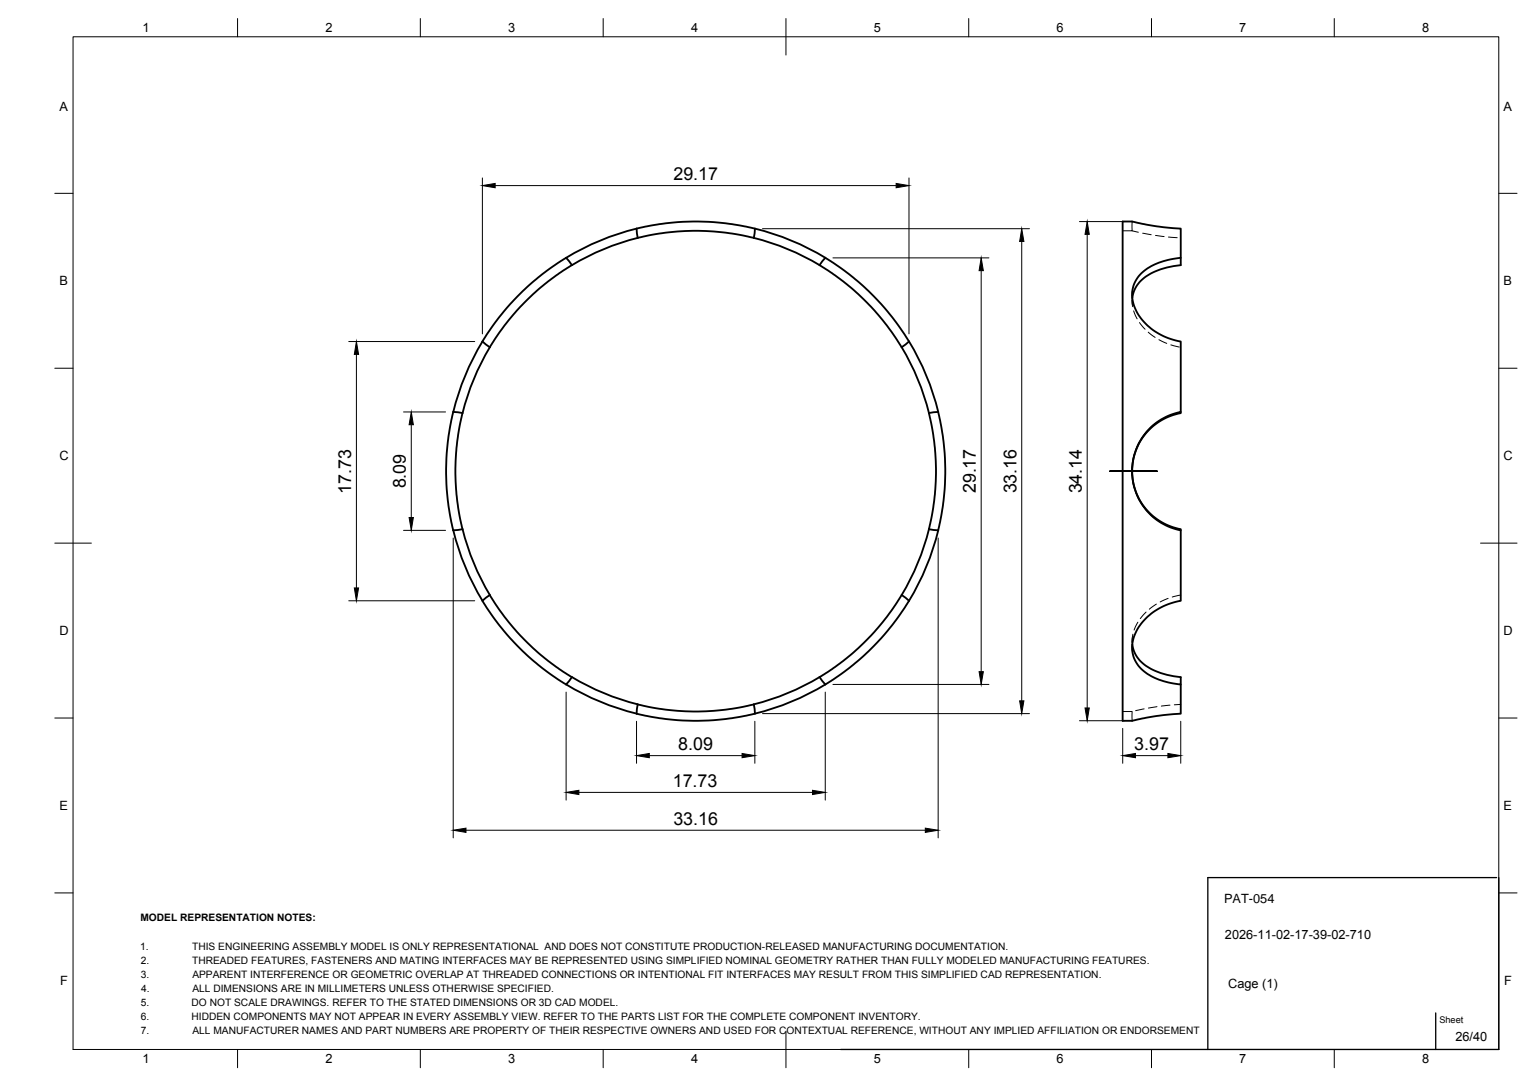
ISO-10303-21;
HEADER;
/* Generated by software containing ST-Developer
 * from STEP Tools, Inc. (www.steptools.com) 
 */

FILE_DESCRIPTION(
/* description */ ('PAT-054'),
/* implementation_level */ '2;1');

FILE_NAME(
/* name */ 'Cage (1).step',
/* time_stamp */ '2026-10-29T16:38:13-07:00',
/* author */ (''),
/* organization */ (''),
/* preprocessor_version */ 'ST-DEVELOPER v20.2',
/* originating_system */ 'Autodesk Translation Framework v15.17.0.0',
/* authorisation */ '');

FILE_SCHEMA (('AUTOMOTIVE_DESIGN { 1 0 10303 214 3 1 1 }'));
ENDSEC;

DATA;
#10=MECHANICAL_DESIGN_GEOMETRIC_PRESENTATION_REPRESENTATION('',(#930),#33981);
#417=B_SPLINE_CURVE_WITH_KNOTS('',3,(#19899,#19900,#19901,#19902,#19903,
#19904,#19905,#19906,#19907,#19908,#19909,#19910,#19911,#19912,#19913,#19914,
#19915,#19916,#19917,#19918,#19919,#19920),.UNSPECIFIED.,.F.,.F.,(4,2,2,
2,2,2,2,2,2,2,4),(0.0789094028588958,0.210573405340968,0.315860108011452,
0.421146810681936,0.522142632548711,0.623138454415485,0.72413427628226,
0.825130098149035,0.930416800819519,1.03570350349,1.16736750597208),
 .UNSPECIFIED.);
#418=B_SPLINE_CURVE_WITH_KNOTS('',3,(#19924,#19925,#19926,#19927,#19928,
#19929,#19930,#19931,#19932,#19933,#19934,#19935,#19936,#19937,#19938,#19939,
#19940,#19941,#19942,#19943,#19944,#19945),.UNSPECIFIED.,.F.,.F.,(4,2,2,
2,2,2,2,2,2,2,4),(0.0774793363974613,0.142088896491891,0.284177792983782,
0.411119756996526,0.514392970548519,0.617666184100513,0.720939397652506,
0.8242126112045,0.951154575217244,1.09324347170913,1.15785303180356),
 .UNSPECIFIED.);
#419=B_SPLINE_CURVE_WITH_KNOTS('',3,(#19951,#19952,#19953,#19954,#19955,
#19956,#19957,#19958,#19959,#19960,#19961,#19962,#19963,#19964,#19965,#19966,
#19967,#19968,#19969,#19970,#19971,#19972),.UNSPECIFIED.,.F.,.F.,(4,2,2,
2,2,2,2,2,2,2,4),(0.0774793363974613,0.142088896491891,0.284177792983782,
0.411119756996525,0.514392970548519,0.617666184100513,0.720939397652506,
0.8242126112045,0.951154575217243,1.09324347170913,1.15785303180356),
 .UNSPECIFIED.);
#420=B_SPLINE_CURVE_WITH_KNOTS('',3,(#19976,#19977,#19978,#19979,#19980,
#19981,#19982,#19983,#19984,#19985,#19986,#19987,#19988,#19989,#19990,#19991,
#19992,#19993,#19994,#19995,#19996,#19997),.UNSPECIFIED.,.F.,.F.,(4,2,2,
2,2,2,2,2,2,2,4),(0.0774793363974614,0.142088896491891,0.284177792983781,
0.411119756996525,0.514392970548519,0.617666184100512,0.720939397652506,
0.824212611204499,0.951154575217243,1.09324347170913,1.15785303180356),
 .UNSPECIFIED.);
#421=B_SPLINE_CURVE_WITH_KNOTS('',3,(#20001,#20002,#20003,#20004,#20005,
#20006,#20007,#20008,#20009,#20010,#20011,#20012),.UNSPECIFIED.,.F.,.F.,
(4,2,2,2,2,4),(0.0774793363974613,0.142088896491891,0.284177792983781,0.411119756996525,
0.514392970548519,0.617666184100512),.UNSPECIFIED.);
#422=B_SPLINE_CURVE_WITH_KNOTS('',3,(#20017,#20018,#20019,#20020,#20021,
#20022,#20023,#20024,#20025,#20026,#20027,#20028),.UNSPECIFIED.,.F.,.F.,
(4,2,2,2,2,4),(0.617666184100512,0.720939397652506,0.824212611204499,0.951154575217243,
1.09324347170913,1.15785303180356),.UNSPECIFIED.);
#423=B_SPLINE_CURVE_WITH_KNOTS('',3,(#20032,#20033,#20034,#20035,#20036,
#20037,#20038,#20039,#20040,#20041,#20042,#20043,#20044,#20045,#20046,#20047,
#20048,#20049,#20050,#20051,#20052,#20053),.UNSPECIFIED.,.F.,.F.,(4,2,2,
2,2,2,2,2,2,2,4),(0.0774793363974613,0.142088896491891,0.284177792983782,
0.411119756996526,0.514392970548519,0.617666184100513,0.720939397652507,
0.8242126112045,0.951154575217245,1.09324347170914,1.15785303180356),
 .UNSPECIFIED.);
#424=B_SPLINE_CURVE_WITH_KNOTS('',3,(#20057,#20058,#20059,#20060,#20061,
#20062,#20063,#20064,#20065,#20066,#20067,#20068,#20069,#20070,#20071,#20072,
#20073,#20074,#20075,#20076,#20077,#20078),.UNSPECIFIED.,.F.,.F.,(4,2,2,
2,2,2,2,2,2,2,4),(0.0774793363974613,0.142088896491891,0.284177792983782,
0.411119756996526,0.514392970548519,0.617666184100513,0.720939397652506,
0.824212611204499,0.951154575217243,1.09324347170913,1.15785303180356),
 .UNSPECIFIED.);
#425=B_SPLINE_CURVE_WITH_KNOTS('',3,(#20082,#20083,#20084,#20085,#20086,
#20087,#20088,#20089,#20090,#20091,#20092,#20093,#20094,#20095,#20096,#20097,
#20098,#20099,#20100,#20101,#20102,#20103),.UNSPECIFIED.,.F.,.F.,(4,2,2,
2,2,2,2,2,2,2,4),(0.0774793363974613,0.142088896491891,0.284177792983782,
0.411119756996526,0.514392970548519,0.617666184100513,0.720939397652506,
0.8242126112045,0.951154575217244,1.09324347170913,1.15785303180356),
 .UNSPECIFIED.);
#426=B_SPLINE_CURVE_WITH_KNOTS('',3,(#20107,#20108,#20109,#20110,#20111,
#20112,#20113,#20114,#20115,#20116,#20117,#20118,#20119,#20120,#20121,#20122,
#20123,#20124,#20125,#20126,#20127,#20128),.UNSPECIFIED.,.F.,.F.,(4,2,2,
2,2,2,2,2,2,2,4),(0.0774793363974613,0.142088896491891,0.284177792983782,
0.411119756996526,0.514392970548519,0.617666184100513,0.720939397652506,
0.8242126112045,0.951154575217243,1.09324347170913,1.15785303180356),
 .UNSPECIFIED.);
#427=B_SPLINE_CURVE_WITH_KNOTS('',3,(#20136,#20137,#20138,#20139,#20140,
#20141,#20142,#20143,#20144,#20145,#20146,#20147,#20148,#20149,#20150,#20151,
#20152,#20153,#20154,#20155,#20156,#20157),.UNSPECIFIED.,.F.,.F.,(4,2,2,
2,2,2,2,2,2,2,4),(0.0789094028588958,0.210573405340968,0.315860108011452,
0.421146810681936,0.522142632548711,0.623138454415485,0.72413427628226,
0.825130098149035,0.930416800819519,1.03570350349,1.16736750597208),
 .UNSPECIFIED.);
#428=B_SPLINE_CURVE_WITH_KNOTS('',3,(#20165,#20166,#20167,#20168,#20169,
#20170,#20171,#20172,#20173,#20174,#20175,#20176,#20177,#20178,#20179,#20180,
#20181,#20182,#20183,#20184,#20185,#20186),.UNSPECIFIED.,.F.,.F.,(4,2,2,
2,2,2,2,2,2,2,4),(0.0789094028588958,0.210573405340969,0.315860108011453,
0.421146810681937,0.522142632548712,0.623138454415486,0.724134276282261,
0.825130098149035,0.930416800819519,1.03570350349,1.16736750597208),
 .UNSPECIFIED.);
#429=B_SPLINE_CURVE_WITH_KNOTS('',3,(#20195,#20196,#20197,#20198,#20199,
#20200,#20201,#20202,#20203,#20204,#20205,#20206),.UNSPECIFIED.,.F.,.F.,
(4,2,2,2,2,4),(0.0789094028588958,0.210573405340968,0.315860108011452,0.421146810681937,
0.522142632548711,0.623138454415486),.UNSPECIFIED.);
#430=B_SPLINE_CURVE_WITH_KNOTS('',3,(#20208,#20209,#20210,#20211,#20212,
#20213,#20214,#20215,#20216,#20217,#20218,#20219),.UNSPECIFIED.,.F.,.F.,
(4,2,2,2,2,4),(0.623138454415486,0.72413427628226,0.825130098149035,0.930416800819519,
1.03570350349,1.16736750597208),.UNSPECIFIED.);
#431=B_SPLINE_CURVE_WITH_KNOTS('',3,(#20226,#20227,#20228,#20229,#20230,
#20231,#20232,#20233,#20234,#20235,#20236,#20237,#20238,#20239,#20240,#20241,
#20242,#20243,#20244,#20245,#20246,#20247),.UNSPECIFIED.,.F.,.F.,(4,2,2,
2,2,2,2,2,2,2,4),(0.0789094028588958,0.210573405340968,0.315860108011452,
0.421146810681936,0.522142632548711,0.623138454415486,0.72413427628226,
0.825130098149035,0.930416800819519,1.03570350349,1.16736750597208),
 .UNSPECIFIED.);
#432=B_SPLINE_CURVE_WITH_KNOTS('',3,(#20255,#20256,#20257,#20258,#20259,
#20260,#20261,#20262,#20263,#20264,#20265,#20266,#20267,#20268,#20269,#20270,
#20271,#20272,#20273,#20274,#20275,#20276),.UNSPECIFIED.,.F.,.F.,(4,2,2,
2,2,2,2,2,2,2,4),(0.0789094028588957,0.210573405340968,0.315860108011452,
0.421146810681936,0.522142632548711,0.623138454415485,0.72413427628226,
0.825130098149035,0.930416800819519,1.03570350349,1.16736750597207),
 .UNSPECIFIED.);
#433=B_SPLINE_CURVE_WITH_KNOTS('',3,(#20284,#20285,#20286,#20287,#20288,
#20289,#20290,#20291,#20292,#20293,#20294,#20295,#20296,#20297,#20298,#20299,
#20300,#20301,#20302,#20303,#20304,#20305),.UNSPECIFIED.,.F.,.F.,(4,2,2,
2,2,2,2,2,2,2,4),(0.0789094028588958,0.210573405340968,0.315860108011452,
0.421146810681936,0.522142632548711,0.623138454415486,0.72413427628226,
0.825130098149035,0.930416800819519,1.03570350349,1.16736750597208),
 .UNSPECIFIED.);
#434=B_SPLINE_CURVE_WITH_KNOTS('',3,(#20314,#20315,#20316,#20317,#20318,
#20319,#20320,#20321,#20322,#20323,#20324,#20325,#20326,#20327,#20328,#20329,
#20330,#20331,#20332,#20333,#20334,#20335),.UNSPECIFIED.,.F.,.F.,(4,2,2,
2,2,2,2,2,2,2,4),(0.0789094028588958,0.210573405340968,0.315860108011452,
0.421146810681936,0.522142632548711,0.623138454415485,0.72413427628226,
0.825130098149035,0.930416800819519,1.03570350349,1.16736750597208),
 .UNSPECIFIED.);
#769=SPHERICAL_SURFACE('',#14058,0.412776);
#770=SPHERICAL_SURFACE('',#14074,0.412776);
#771=SPHERICAL_SURFACE('',#14079,0.412776);
#772=SPHERICAL_SURFACE('',#14084,0.412776);
#773=SPHERICAL_SURFACE('',#14089,0.412776);
#774=SPHERICAL_SURFACE('',#14094,0.412776);
#775=SPHERICAL_SURFACE('',#14099,0.412776);
#776=SPHERICAL_SURFACE('',#14107,0.412776);
#828=SHAPE_REPRESENTATION_RELATIONSHIP('SRR','None',#34203,#872);
#872=ADVANCED_BREP_SHAPE_REPRESENTATION('',(#989),#33951);
#930=STYLED_ITEM('',(#34517),#989);
#989=MANIFOLD_SOLID_BREP('Continuous crown cage',#13041);
#1141=FACE_BOUND('',#2670,.T.);
#1331=PLANE('',#14071);
#1332=PLANE('',#14076);
#1333=PLANE('',#14081);
#1334=PLANE('',#14086);
#1335=PLANE('',#14091);
#1336=PLANE('',#14096);
#1337=PLANE('',#14105);
#1338=PLANE('',#14109);
#1339=PLANE('',#14110);
#1800=FACE_OUTER_BOUND('',#2652,.T.);
#1801=FACE_OUTER_BOUND('',#2653,.T.);
#1802=FACE_OUTER_BOUND('',#2654,.T.);
#1803=FACE_OUTER_BOUND('',#2655,.T.);
#1804=FACE_OUTER_BOUND('',#2656,.T.);
#1805=FACE_OUTER_BOUND('',#2657,.T.);
#1806=FACE_OUTER_BOUND('',#2658,.T.);
#1807=FACE_OUTER_BOUND('',#2659,.T.);
#1808=FACE_OUTER_BOUND('',#2660,.T.);
#1809=FACE_OUTER_BOUND('',#2661,.T.);
#1810=FACE_OUTER_BOUND('',#2662,.T.);
#1811=FACE_OUTER_BOUND('',#2663,.T.);
#1812=FACE_OUTER_BOUND('',#2664,.T.);
#1813=FACE_OUTER_BOUND('',#2665,.T.);
#1814=FACE_OUTER_BOUND('',#2666,.T.);
#1815=FACE_OUTER_BOUND('',#2667,.T.);
#1816=FACE_OUTER_BOUND('',#2668,.T.);
#1817=FACE_OUTER_BOUND('',#2669,.T.);
#1818=FACE_OUTER_BOUND('',#2671,.T.);
#2652=EDGE_LOOP('',(#9505,#9506,#9507,#9508));
#2653=EDGE_LOOP('',(#9509,#9510,#9511,#9512,#9513,#9514,#9515,#9516,#9517,
#9518,#9519,#9520,#9521,#9522,#9523,#9524,#9525,#9526,#9527,#9528));
#2654=EDGE_LOOP('',(#9529,#9530,#9531,#9532));
#2655=EDGE_LOOP('',(#9533,#9534,#9535,#9536));
#2656=EDGE_LOOP('',(#9537,#9538,#9539,#9540));
#2657=EDGE_LOOP('',(#9541,#9542,#9543,#9544));
#2658=EDGE_LOOP('',(#9545,#9546,#9547,#9548));
#2659=EDGE_LOOP('',(#9549,#9550,#9551,#9552,#9553,#9554));
#2660=EDGE_LOOP('',(#9555,#9556,#9557,#9558));
#2661=EDGE_LOOP('',(#9559,#9560,#9561,#9562));
#2662=EDGE_LOOP('',(#9563,#9564,#9565,#9566));
#2663=EDGE_LOOP('',(#9567,#9568,#9569,#9570));
#2664=EDGE_LOOP('',(#9571,#9572,#9573,#9574));
#2665=EDGE_LOOP('',(#9575,#9576,#9577,#9578));
#2666=EDGE_LOOP('',(#9579,#9580,#9581,#9582,#9583,#9584,#9585,#9586,#9587,
#9588,#9589,#9590,#9591,#9592,#9593,#9594,#9595,#9596,#9597,#9598));
#2667=EDGE_LOOP('',(#9599,#9600,#9601,#9602));
#2668=EDGE_LOOP('',(#9603,#9604,#9605,#9606));
#2669=EDGE_LOOP('',(#9607));
#2670=EDGE_LOOP('',(#9608));
#2671=EDGE_LOOP('',(#9609,#9610,#9611,#9612));
#3484=LINE('',#20014,#4418);
#3485=LINE('',#20310,#4419);
#4418=VECTOR('',#16149,1.706752);
#4419=VECTOR('',#16226,1.643248);
#5352=CIRCLE('',#14059,0.405071403305639);
#5353=CIRCLE('',#14060,0.405071403305639);
#5354=CIRCLE('',#14062,1.706752);
#5355=CIRCLE('',#14063,1.706752);
#5356=CIRCLE('',#14064,1.706752);
#5357=CIRCLE('',#14065,1.706752);
#5358=CIRCLE('',#14066,1.706752);
#5359=CIRCLE('',#14067,1.706752);
#5360=CIRCLE('',#14068,1.706752);
#5361=CIRCLE('',#14069,1.706752);
#5362=CIRCLE('',#14070,1.706752);
#5363=CIRCLE('',#14072,1.643248);
#5364=CIRCLE('',#14073,0.405071403305639);
#5365=CIRCLE('',#14075,0.405071403305639);
#5366=CIRCLE('',#14077,1.643248);
#5367=CIRCLE('',#14078,0.405071403305639);
#5368=CIRCLE('',#14080,0.405071403305639);
#5369=CIRCLE('',#14082,1.643248);
#5370=CIRCLE('',#14083,0.405071403305639);
#5371=CIRCLE('',#14085,0.405071403305639);
#5372=CIRCLE('',#14087,1.643248);
#5373=CIRCLE('',#14088,0.405071403305639);
#5374=CIRCLE('',#14090,0.405071403305639);
#5375=CIRCLE('',#14092,1.643248);
#5376=CIRCLE('',#14093,0.405071403305639);
#5377=CIRCLE('',#14095,0.405071403305639);
#5378=CIRCLE('',#14097,1.643248);
#5379=CIRCLE('',#14098,0.405071403305639);
#5380=CIRCLE('',#14100,0.405071403305639);
#5381=CIRCLE('',#14102,1.643248);
#5382=CIRCLE('',#14103,1.643248);
#5383=CIRCLE('',#14104,1.643248);
#5384=CIRCLE('',#14106,0.405071403305639);
#5385=CIRCLE('',#14108,0.405071403305639);
#5926=VERTEX_POINT('',#19897);
#5927=VERTEX_POINT('',#19898);
#5928=VERTEX_POINT('',#19921);
#5929=VERTEX_POINT('',#19923);
#5930=VERTEX_POINT('',#19948);
#5931=VERTEX_POINT('',#19950);
#5932=VERTEX_POINT('',#19973);
#5933=VERTEX_POINT('',#19975);
#5934=VERTEX_POINT('',#19998);
#5935=VERTEX_POINT('',#20000);
#5936=VERTEX_POINT('',#20013);
#5937=VERTEX_POINT('',#20016);
#5938=VERTEX_POINT('',#20029);
#5939=VERTEX_POINT('',#20031);
#5940=VERTEX_POINT('',#20054);
#5941=VERTEX_POINT('',#20056);
#5942=VERTEX_POINT('',#20079);
#5943=VERTEX_POINT('',#20081);
#5944=VERTEX_POINT('',#20104);
#5945=VERTEX_POINT('',#20106);
#5946=VERTEX_POINT('',#20131);
#5947=VERTEX_POINT('',#20135);
#5948=VERTEX_POINT('',#20160);
#5949=VERTEX_POINT('',#20164);
#5950=VERTEX_POINT('',#20189);
#5951=VERTEX_POINT('',#20193);
#5952=VERTEX_POINT('',#20194);
#5953=VERTEX_POINT('',#20221);
#5954=VERTEX_POINT('',#20225);
#5955=VERTEX_POINT('',#20250);
#5956=VERTEX_POINT('',#20254);
#5957=VERTEX_POINT('',#20279);
#5958=VERTEX_POINT('',#20283);
#5959=VERTEX_POINT('',#20308);
#5960=VERTEX_POINT('',#20311);
#5961=VERTEX_POINT('',#20313);
#7252=EDGE_CURVE('',#5926,#5927,#417,.T.);
#7253=EDGE_CURVE('',#5928,#5926,#5352,.T.);
#7254=EDGE_CURVE('',#5929,#5928,#418,.T.);
#7255=EDGE_CURVE('',#5927,#5929,#5353,.T.);
#7256=EDGE_CURVE('',#5930,#5928,#5354,.T.);
#7257=EDGE_CURVE('',#5930,#5931,#419,.T.);
#7258=EDGE_CURVE('',#5932,#5931,#5355,.T.);
#7259=EDGE_CURVE('',#5932,#5933,#420,.T.);
#7260=EDGE_CURVE('',#5934,#5933,#5356,.T.);
#7261=EDGE_CURVE('',#5934,#5935,#421,.T.);
#7262=EDGE_CURVE('',#5935,#5936,#3484,.T.);
#7263=EDGE_CURVE('',#5936,#5936,#5357,.T.);
#7264=EDGE_CURVE('',#5935,#5937,#422,.T.);
#7265=EDGE_CURVE('',#5938,#5937,#5358,.T.);
#7266=EDGE_CURVE('',#5938,#5939,#423,.T.);
#7267=EDGE_CURVE('',#5940,#5939,#5359,.T.);
#7268=EDGE_CURVE('',#5940,#5941,#424,.T.);
#7269=EDGE_CURVE('',#5942,#5941,#5360,.T.);
#7270=EDGE_CURVE('',#5942,#5943,#425,.T.);
#7271=EDGE_CURVE('',#5944,#5943,#5361,.T.);
#7272=EDGE_CURVE('',#5944,#5945,#426,.T.);
#7273=EDGE_CURVE('',#5929,#5945,#5362,.T.);
#7274=EDGE_CURVE('',#5926,#5946,#5363,.T.);
#7275=EDGE_CURVE('',#5946,#5930,#5364,.T.);
#7276=EDGE_CURVE('',#5947,#5946,#427,.T.);
#7277=EDGE_CURVE('',#5931,#5947,#5365,.T.);
#7278=EDGE_CURVE('',#5947,#5948,#5366,.T.);
#7279=EDGE_CURVE('',#5948,#5932,#5367,.T.);
#7280=EDGE_CURVE('',#5949,#5948,#428,.T.);
#7281=EDGE_CURVE('',#5933,#5949,#5368,.T.);
#7282=EDGE_CURVE('',#5949,#5950,#5369,.T.);
#7283=EDGE_CURVE('',#5950,#5934,#5370,.T.);
#7284=EDGE_CURVE('',#5951,#5952,#429,.T.);
#7285=EDGE_CURVE('',#5937,#5951,#5371,.T.);
#7286=EDGE_CURVE('',#5952,#5950,#430,.T.);
#7287=EDGE_CURVE('',#5951,#5953,#5372,.T.);
#7288=EDGE_CURVE('',#5953,#5938,#5373,.T.);
#7289=EDGE_CURVE('',#5954,#5953,#431,.T.);
#7290=EDGE_CURVE('',#5939,#5954,#5374,.T.);
#7291=EDGE_CURVE('',#5954,#5955,#5375,.T.);
#7292=EDGE_CURVE('',#5955,#5940,#5376,.T.);
#7293=EDGE_CURVE('',#5956,#5955,#432,.T.);
#7294=EDGE_CURVE('',#5941,#5956,#5377,.T.);
#7295=EDGE_CURVE('',#5956,#5957,#5378,.T.);
#7296=EDGE_CURVE('',#5957,#5942,#5379,.T.);
#7297=EDGE_CURVE('',#5958,#5957,#433,.T.);
#7298=EDGE_CURVE('',#5943,#5958,#5380,.T.);
#7299=EDGE_CURVE('',#5959,#5959,#5381,.T.);
#7300=EDGE_CURVE('',#5959,#5952,#3485,.T.);
#7301=EDGE_CURVE('',#5960,#5927,#5382,.T.);
#7302=EDGE_CURVE('',#5960,#5961,#434,.T.);
#7303=EDGE_CURVE('',#5958,#5961,#5383,.T.);
#7304=EDGE_CURVE('',#5945,#5960,#5384,.T.);
#7305=EDGE_CURVE('',#5961,#5944,#5385,.T.);
#9505=ORIENTED_EDGE('',*,*,#7252,.F.);
#9506=ORIENTED_EDGE('',*,*,#7253,.F.);
#9507=ORIENTED_EDGE('',*,*,#7254,.F.);
#9508=ORIENTED_EDGE('',*,*,#7255,.F.);
#9509=ORIENTED_EDGE('',*,*,#7254,.T.);
#9510=ORIENTED_EDGE('',*,*,#7256,.F.);
#9511=ORIENTED_EDGE('',*,*,#7257,.T.);
#9512=ORIENTED_EDGE('',*,*,#7258,.F.);
#9513=ORIENTED_EDGE('',*,*,#7259,.T.);
#9514=ORIENTED_EDGE('',*,*,#7260,.F.);
#9515=ORIENTED_EDGE('',*,*,#7261,.T.);
#9516=ORIENTED_EDGE('',*,*,#7262,.T.);
#9517=ORIENTED_EDGE('',*,*,#7263,.F.);
#9518=ORIENTED_EDGE('',*,*,#7262,.F.);
#9519=ORIENTED_EDGE('',*,*,#7264,.T.);
#9520=ORIENTED_EDGE('',*,*,#7265,.F.);
#9521=ORIENTED_EDGE('',*,*,#7266,.T.);
#9522=ORIENTED_EDGE('',*,*,#7267,.F.);
#9523=ORIENTED_EDGE('',*,*,#7268,.T.);
#9524=ORIENTED_EDGE('',*,*,#7269,.F.);
#9525=ORIENTED_EDGE('',*,*,#7270,.T.);
#9526=ORIENTED_EDGE('',*,*,#7271,.F.);
#9527=ORIENTED_EDGE('',*,*,#7272,.T.);
#9528=ORIENTED_EDGE('',*,*,#7273,.F.);
#9529=ORIENTED_EDGE('',*,*,#7253,.T.);
#9530=ORIENTED_EDGE('',*,*,#7274,.T.);
#9531=ORIENTED_EDGE('',*,*,#7275,.T.);
#9532=ORIENTED_EDGE('',*,*,#7256,.T.);
#9533=ORIENTED_EDGE('',*,*,#7276,.F.);
#9534=ORIENTED_EDGE('',*,*,#7277,.F.);
#9535=ORIENTED_EDGE('',*,*,#7257,.F.);
#9536=ORIENTED_EDGE('',*,*,#7275,.F.);
#9537=ORIENTED_EDGE('',*,*,#7277,.T.);
#9538=ORIENTED_EDGE('',*,*,#7278,.T.);
#9539=ORIENTED_EDGE('',*,*,#7279,.T.);
#9540=ORIENTED_EDGE('',*,*,#7258,.T.);
#9541=ORIENTED_EDGE('',*,*,#7280,.F.);
#9542=ORIENTED_EDGE('',*,*,#7281,.F.);
#9543=ORIENTED_EDGE('',*,*,#7259,.F.);
#9544=ORIENTED_EDGE('',*,*,#7279,.F.);
#9545=ORIENTED_EDGE('',*,*,#7281,.T.);
#9546=ORIENTED_EDGE('',*,*,#7282,.T.);
#9547=ORIENTED_EDGE('',*,*,#7283,.T.);
#9548=ORIENTED_EDGE('',*,*,#7260,.T.);
#9549=ORIENTED_EDGE('',*,*,#7284,.F.);
#9550=ORIENTED_EDGE('',*,*,#7285,.F.);
#9551=ORIENTED_EDGE('',*,*,#7264,.F.);
#9552=ORIENTED_EDGE('',*,*,#7261,.F.);
#9553=ORIENTED_EDGE('',*,*,#7283,.F.);
#9554=ORIENTED_EDGE('',*,*,#7286,.F.);
#9555=ORIENTED_EDGE('',*,*,#7285,.T.);
#9556=ORIENTED_EDGE('',*,*,#7287,.T.);
#9557=ORIENTED_EDGE('',*,*,#7288,.T.);
#9558=ORIENTED_EDGE('',*,*,#7265,.T.);
#9559=ORIENTED_EDGE('',*,*,#7289,.F.);
#9560=ORIENTED_EDGE('',*,*,#7290,.F.);
#9561=ORIENTED_EDGE('',*,*,#7266,.F.);
#9562=ORIENTED_EDGE('',*,*,#7288,.F.);
#9563=ORIENTED_EDGE('',*,*,#7290,.T.);
#9564=ORIENTED_EDGE('',*,*,#7291,.T.);
#9565=ORIENTED_EDGE('',*,*,#7292,.T.);
#9566=ORIENTED_EDGE('',*,*,#7267,.T.);
#9567=ORIENTED_EDGE('',*,*,#7293,.F.);
#9568=ORIENTED_EDGE('',*,*,#7294,.F.);
#9569=ORIENTED_EDGE('',*,*,#7268,.F.);
#9570=ORIENTED_EDGE('',*,*,#7292,.F.);
#9571=ORIENTED_EDGE('',*,*,#7294,.T.);
#9572=ORIENTED_EDGE('',*,*,#7295,.T.);
#9573=ORIENTED_EDGE('',*,*,#7296,.T.);
#9574=ORIENTED_EDGE('',*,*,#7269,.T.);
#9575=ORIENTED_EDGE('',*,*,#7270,.F.);
#9576=ORIENTED_EDGE('',*,*,#7296,.F.);
#9577=ORIENTED_EDGE('',*,*,#7297,.F.);
#9578=ORIENTED_EDGE('',*,*,#7298,.F.);
#9579=ORIENTED_EDGE('',*,*,#7299,.F.);
#9580=ORIENTED_EDGE('',*,*,#7300,.T.);
#9581=ORIENTED_EDGE('',*,*,#7286,.T.);
#9582=ORIENTED_EDGE('',*,*,#7282,.F.);
#9583=ORIENTED_EDGE('',*,*,#7280,.T.);
#9584=ORIENTED_EDGE('',*,*,#7278,.F.);
#9585=ORIENTED_EDGE('',*,*,#7276,.T.);
#9586=ORIENTED_EDGE('',*,*,#7274,.F.);
#9587=ORIENTED_EDGE('',*,*,#7252,.T.);
#9588=ORIENTED_EDGE('',*,*,#7301,.F.);
#9589=ORIENTED_EDGE('',*,*,#7302,.T.);
#9590=ORIENTED_EDGE('',*,*,#7303,.F.);
#9591=ORIENTED_EDGE('',*,*,#7297,.T.);
#9592=ORIENTED_EDGE('',*,*,#7295,.F.);
#9593=ORIENTED_EDGE('',*,*,#7293,.T.);
#9594=ORIENTED_EDGE('',*,*,#7291,.F.);
#9595=ORIENTED_EDGE('',*,*,#7289,.T.);
#9596=ORIENTED_EDGE('',*,*,#7287,.F.);
#9597=ORIENTED_EDGE('',*,*,#7284,.T.);
#9598=ORIENTED_EDGE('',*,*,#7300,.F.);
#9599=ORIENTED_EDGE('',*,*,#7255,.T.);
#9600=ORIENTED_EDGE('',*,*,#7273,.T.);
#9601=ORIENTED_EDGE('',*,*,#7304,.T.);
#9602=ORIENTED_EDGE('',*,*,#7301,.T.);
#9603=ORIENTED_EDGE('',*,*,#7272,.F.);
#9604=ORIENTED_EDGE('',*,*,#7305,.F.);
#9605=ORIENTED_EDGE('',*,*,#7302,.F.);
#9606=ORIENTED_EDGE('',*,*,#7304,.F.);
#9607=ORIENTED_EDGE('',*,*,#7263,.T.);
#9608=ORIENTED_EDGE('',*,*,#7299,.T.);
#9609=ORIENTED_EDGE('',*,*,#7298,.T.);
#9610=ORIENTED_EDGE('',*,*,#7303,.T.);
#9611=ORIENTED_EDGE('',*,*,#7305,.T.);
#9612=ORIENTED_EDGE('',*,*,#7271,.T.);
#12067=CYLINDRICAL_SURFACE('',#14061,1.706752);
#12068=CYLINDRICAL_SURFACE('',#14101,1.643248);
#12512=ADVANCED_FACE('',(#1800),#769,.F.);
#12513=ADVANCED_FACE('',(#1801),#12067,.T.);
#12514=ADVANCED_FACE('',(#1802),#1331,.T.);
#12515=ADVANCED_FACE('',(#1803),#770,.F.);
#12516=ADVANCED_FACE('',(#1804),#1332,.T.);
#12517=ADVANCED_FACE('',(#1805),#771,.F.);
#12518=ADVANCED_FACE('',(#1806),#1333,.T.);
#12519=ADVANCED_FACE('',(#1807),#772,.F.);
#12520=ADVANCED_FACE('',(#1808),#1334,.T.);
#12521=ADVANCED_FACE('',(#1809),#773,.F.);
#12522=ADVANCED_FACE('',(#1810),#1335,.T.);
#12523=ADVANCED_FACE('',(#1811),#774,.F.);
#12524=ADVANCED_FACE('',(#1812),#1336,.T.);
#12525=ADVANCED_FACE('',(#1813),#775,.F.);
#12526=ADVANCED_FACE('',(#1814),#12068,.F.);
#12527=ADVANCED_FACE('',(#1815),#1337,.T.);
#12528=ADVANCED_FACE('',(#1816),#776,.F.);
#12529=ADVANCED_FACE('',(#1817,#1141),#1338,.T.);
#12530=ADVANCED_FACE('',(#1818),#1339,.T.);
#13041=CLOSED_SHELL('',(#12512,#12513,#12514,#12515,#12516,#12517,#12518,
#12519,#12520,#12521,#12522,#12523,#12524,#12525,#12526,#12527,#12528,#12529,
#12530));
#14057=AXIS2_PLACEMENT_3D('',#19895,#16133,#16134);
#14058=AXIS2_PLACEMENT_3D('',#19896,#16135,#16136);
#14059=AXIS2_PLACEMENT_3D('',#19922,#16137,#16138);
#14060=AXIS2_PLACEMENT_3D('',#19946,#16139,#16140);
#14061=AXIS2_PLACEMENT_3D('',#19947,#16141,#16142);
#14062=AXIS2_PLACEMENT_3D('',#19949,#16143,#16144);
#14063=AXIS2_PLACEMENT_3D('',#19974,#16145,#16146);
#14064=AXIS2_PLACEMENT_3D('',#19999,#16147,#16148);
#14065=AXIS2_PLACEMENT_3D('',#20015,#16150,#16151);
#14066=AXIS2_PLACEMENT_3D('',#20030,#16152,#16153);
#14067=AXIS2_PLACEMENT_3D('',#20055,#16154,#16155);
#14068=AXIS2_PLACEMENT_3D('',#20080,#16156,#16157);
#14069=AXIS2_PLACEMENT_3D('',#20105,#16158,#16159);
#14070=AXIS2_PLACEMENT_3D('',#20129,#16160,#16161);
#14071=AXIS2_PLACEMENT_3D('',#20130,#16162,#16163);
#14072=AXIS2_PLACEMENT_3D('',#20132,#16164,#16165);
#14073=AXIS2_PLACEMENT_3D('',#20133,#16166,#16167);
#14074=AXIS2_PLACEMENT_3D('',#20134,#16168,#16169);
#14075=AXIS2_PLACEMENT_3D('',#20158,#16170,#16171);
#14076=AXIS2_PLACEMENT_3D('',#20159,#16172,#16173);
#14077=AXIS2_PLACEMENT_3D('',#20161,#16174,#16175);
#14078=AXIS2_PLACEMENT_3D('',#20162,#16176,#16177);
#14079=AXIS2_PLACEMENT_3D('',#20163,#16178,#16179);
#14080=AXIS2_PLACEMENT_3D('',#20187,#16180,#16181);
#14081=AXIS2_PLACEMENT_3D('',#20188,#16182,#16183);
#14082=AXIS2_PLACEMENT_3D('',#20190,#16184,#16185);
#14083=AXIS2_PLACEMENT_3D('',#20191,#16186,#16187);
#14084=AXIS2_PLACEMENT_3D('',#20192,#16188,#16189);
#14085=AXIS2_PLACEMENT_3D('',#20207,#16190,#16191);
#14086=AXIS2_PLACEMENT_3D('',#20220,#16192,#16193);
#14087=AXIS2_PLACEMENT_3D('',#20222,#16194,#16195);
#14088=AXIS2_PLACEMENT_3D('',#20223,#16196,#16197);
#14089=AXIS2_PLACEMENT_3D('',#20224,#16198,#16199);
#14090=AXIS2_PLACEMENT_3D('',#20248,#16200,#16201);
#14091=AXIS2_PLACEMENT_3D('',#20249,#16202,#16203);
#14092=AXIS2_PLACEMENT_3D('',#20251,#16204,#16205);
#14093=AXIS2_PLACEMENT_3D('',#20252,#16206,#16207);
#14094=AXIS2_PLACEMENT_3D('',#20253,#16208,#16209);
#14095=AXIS2_PLACEMENT_3D('',#20277,#16210,#16211);
#14096=AXIS2_PLACEMENT_3D('',#20278,#16212,#16213);
#14097=AXIS2_PLACEMENT_3D('',#20280,#16214,#16215);
#14098=AXIS2_PLACEMENT_3D('',#20281,#16216,#16217);
#14099=AXIS2_PLACEMENT_3D('',#20282,#16218,#16219);
#14100=AXIS2_PLACEMENT_3D('',#20306,#16220,#16221);
#14101=AXIS2_PLACEMENT_3D('',#20307,#16222,#16223);
#14102=AXIS2_PLACEMENT_3D('',#20309,#16224,#16225);
#14103=AXIS2_PLACEMENT_3D('',#20312,#16227,#16228);
#14104=AXIS2_PLACEMENT_3D('',#20336,#16229,#16230);
#14105=AXIS2_PLACEMENT_3D('',#20337,#16231,#16232);
#14106=AXIS2_PLACEMENT_3D('',#20338,#16233,#16234);
#14107=AXIS2_PLACEMENT_3D('',#20339,#16235,#16236);
#14108=AXIS2_PLACEMENT_3D('',#20340,#16237,#16238);
#14109=AXIS2_PLACEMENT_3D('',#20341,#16239,#16240);
#14110=AXIS2_PLACEMENT_3D('',#20342,#16241,#16242);
#16133=DIRECTION('axis',(0.,0.,1.));
#16134=DIRECTION('refdir',(1.,0.,0.));
#16135=DIRECTION('center_axis',(0.,0.,1.));
#16136=DIRECTION('ref_axis',(1.,0.,0.));
#16137=DIRECTION('center_axis',(0.,-1.,0.));
#16138=DIRECTION('ref_axis',(0.,0.,-1.));
#16139=DIRECTION('center_axis',(0.,-1.,0.));
#16140=DIRECTION('ref_axis',(0.,0.,-1.));
#16141=DIRECTION('center_axis',(0.,1.,0.));
#16142=DIRECTION('ref_axis',(1.,0.,0.));
#16143=DIRECTION('center_axis',(0.,1.,0.));
#16144=DIRECTION('ref_axis',(1.,0.,0.));
#16145=DIRECTION('center_axis',(0.,1.,0.));
#16146=DIRECTION('ref_axis',(1.,0.,0.));
#16147=DIRECTION('center_axis',(0.,1.,0.));
#16148=DIRECTION('ref_axis',(1.,0.,0.));
#16149=DIRECTION('',(0.,-1.,0.));
#16150=DIRECTION('center_axis',(0.,-1.,0.));
#16151=DIRECTION('ref_axis',(1.,0.,0.));
#16152=DIRECTION('center_axis',(0.,1.,0.));
#16153=DIRECTION('ref_axis',(1.,0.,0.));
#16154=DIRECTION('center_axis',(0.,1.,0.));
#16155=DIRECTION('ref_axis',(1.,0.,0.));
#16156=DIRECTION('center_axis',(0.,1.,0.));
#16157=DIRECTION('ref_axis',(1.,0.,0.));
#16158=DIRECTION('center_axis',(0.,1.,0.));
#16159=DIRECTION('ref_axis',(1.,0.,0.));
#16160=DIRECTION('center_axis',(0.,1.,0.));
#16161=DIRECTION('ref_axis',(1.,0.,0.));
#16162=DIRECTION('center_axis',(0.,1.,0.));
#16163=DIRECTION('ref_axis',(1.,0.,0.));
#16164=DIRECTION('center_axis',(0.,-1.,0.));
#16165=DIRECTION('ref_axis',(1.,0.,0.));
#16166=DIRECTION('center_axis',(0.,-1.,0.));
#16167=DIRECTION('ref_axis',(0.,0.,-1.));
#16168=DIRECTION('center_axis',(6.12323399573677E-17,0.,1.));
#16169=DIRECTION('ref_axis',(1.,0.,0.));
#16170=DIRECTION('center_axis',(0.,-1.,0.));
#16171=DIRECTION('ref_axis',(0.,0.,-1.));
#16172=DIRECTION('center_axis',(0.,1.,0.));
#16173=DIRECTION('ref_axis',(1.,0.,0.));
#16174=DIRECTION('center_axis',(0.,-1.,0.));
#16175=DIRECTION('ref_axis',(1.,0.,0.));
#16176=DIRECTION('center_axis',(0.,-1.,0.));
#16177=DIRECTION('ref_axis',(0.,0.,-1.));
#16178=DIRECTION('center_axis',(0.,0.,1.));
#16179=DIRECTION('ref_axis',(1.,0.,0.));
#16180=DIRECTION('center_axis',(0.,-1.,0.));
#16181=DIRECTION('ref_axis',(0.,0.,-1.));
#16182=DIRECTION('center_axis',(0.,1.,0.));
#16183=DIRECTION('ref_axis',(1.,0.,0.));
#16184=DIRECTION('center_axis',(0.,-1.,0.));
#16185=DIRECTION('ref_axis',(1.,0.,0.));
#16186=DIRECTION('center_axis',(0.,-1.,0.));
#16187=DIRECTION('ref_axis',(0.,0.,-1.));
#16188=DIRECTION('center_axis',(0.,0.,1.));
#16189=DIRECTION('ref_axis',(1.,0.,0.));
#16190=DIRECTION('center_axis',(0.,-1.,0.));
#16191=DIRECTION('ref_axis',(0.,0.,-1.));
#16192=DIRECTION('center_axis',(0.,1.,0.));
#16193=DIRECTION('ref_axis',(1.,0.,0.));
#16194=DIRECTION('center_axis',(0.,-1.,0.));
#16195=DIRECTION('ref_axis',(1.,0.,0.));
#16196=DIRECTION('center_axis',(0.,-1.,0.));
#16197=DIRECTION('ref_axis',(0.,0.,-1.));
#16198=DIRECTION('center_axis',(0.,0.,1.));
#16199=DIRECTION('ref_axis',(1.,0.,0.));
#16200=DIRECTION('center_axis',(0.,-1.,0.));
#16201=DIRECTION('ref_axis',(0.,0.,-1.));
#16202=DIRECTION('center_axis',(0.,1.,0.));
#16203=DIRECTION('ref_axis',(1.,0.,0.));
#16204=DIRECTION('center_axis',(0.,-1.,0.));
#16205=DIRECTION('ref_axis',(1.,0.,0.));
#16206=DIRECTION('center_axis',(0.,-1.,0.));
#16207=DIRECTION('ref_axis',(0.,0.,-1.));
#16208=DIRECTION('center_axis',(6.12323399573676E-17,0.,1.));
#16209=DIRECTION('ref_axis',(1.,0.,0.));
#16210=DIRECTION('center_axis',(0.,-1.,0.));
#16211=DIRECTION('ref_axis',(0.,0.,-1.));
#16212=DIRECTION('center_axis',(0.,1.,0.));
#16213=DIRECTION('ref_axis',(1.,0.,0.));
#16214=DIRECTION('center_axis',(0.,-1.,0.));
#16215=DIRECTION('ref_axis',(1.,0.,0.));
#16216=DIRECTION('center_axis',(0.,-1.,0.));
#16217=DIRECTION('ref_axis',(0.,0.,-1.));
#16218=DIRECTION('center_axis',(0.,0.,1.));
#16219=DIRECTION('ref_axis',(1.,0.,0.));
#16220=DIRECTION('center_axis',(0.,-1.,0.));
#16221=DIRECTION('ref_axis',(0.,0.,-1.));
#16222=DIRECTION('center_axis',(0.,1.,0.));
#16223=DIRECTION('ref_axis',(1.,0.,0.));
#16224=DIRECTION('center_axis',(0.,1.,0.));
#16225=DIRECTION('ref_axis',(1.,0.,0.));
#16226=DIRECTION('',(0.,1.,0.));
#16227=DIRECTION('center_axis',(0.,-1.,0.));
#16228=DIRECTION('ref_axis',(1.,0.,0.));
#16229=DIRECTION('center_axis',(0.,-1.,0.));
#16230=DIRECTION('ref_axis',(1.,0.,0.));
#16231=DIRECTION('center_axis',(0.,1.,0.));
#16232=DIRECTION('ref_axis',(1.,0.,0.));
#16233=DIRECTION('center_axis',(0.,-1.,0.));
#16234=DIRECTION('ref_axis',(0.,0.,-1.));
#16235=DIRECTION('center_axis',(0.,0.,1.));
#16236=DIRECTION('ref_axis',(1.,0.,0.));
#16237=DIRECTION('center_axis',(0.,-1.,0.));
#16238=DIRECTION('ref_axis',(0.,0.,-1.));
#16239=DIRECTION('center_axis',(0.,-1.,0.));
#16240=DIRECTION('ref_axis',(-1.,0.,0.));
#16241=DIRECTION('center_axis',(0.,1.,0.));
#16242=DIRECTION('ref_axis',(1.,0.,0.));
#19895=CARTESIAN_POINT('',(0.,0.,0.));
#19896=CARTESIAN_POINT('Origin',(1.18440385848747,0.,1.18440385848747));
#19897=CARTESIAN_POINT('',(0.846804978391753,-0.07938,1.40825612658882));
#19898=CARTESIAN_POINT('',(1.40825612658882,-0.07938,0.846804978391754));
#19899=CARTESIAN_POINT('Ctrl Pts',(0.846804978391752,-0.0793800000000001,
1.40825612658882));
#19900=CARTESIAN_POINT('Ctrl Pts',(0.854205272175554,-0.123401821157026,
1.40380622184538));
#19901=CARTESIAN_POINT('Ctrl Pts',(0.867957148219441,-0.166543350814306,
1.39550172959303));
#19902=CARTESIAN_POINT('Ctrl Pts',(0.902193646979982,-0.237231147975234,
1.3735491215176));
#19903=CARTESIAN_POINT('Ctrl Pts',(0.920778333482564,-0.266264900654909,
1.36127834356734));
#19904=CARTESIAN_POINT('Ctrl Pts',(0.962485392528369,-0.317195968905306,
1.33211611256184));
#19905=CARTESIAN_POINT('Ctrl Pts',(0.985600426557816,-0.33909093068465,
1.31521005565926));
#19906=CARTESIAN_POINT('Ctrl Pts',(1.03253285680459,-0.373586846396559,
1.27866649102984));
#19907=CARTESIAN_POINT('Ctrl Pts',(1.05871835910697,-0.388086240756494,
1.25722555095714));
#19908=CARTESIAN_POINT('Ctrl Pts',(1.11153475808518,-0.407068917407805,
1.2107812086231));
#19909=CARTESIAN_POINT('Ctrl Pts',(1.13814686046673,-0.411552957311693,
1.18575674747573));
#19910=CARTESIAN_POINT('Ctrl Pts',(1.18575674747573,-0.411552957311693,
1.13814686046673));
#19911=CARTESIAN_POINT('Ctrl Pts',(1.2107812086231,-0.407068917407805,1.11153475808518));
#19912=CARTESIAN_POINT('Ctrl Pts',(1.25722555095713,-0.388086240756494,
1.05871835910697));
#19913=CARTESIAN_POINT('Ctrl Pts',(1.27866649102984,-0.373586846396559,
1.03253285680459));
#19914=CARTESIAN_POINT('Ctrl Pts',(1.31521005565926,-0.33909093068465,0.985600426557816));
#19915=CARTESIAN_POINT('Ctrl Pts',(1.33211611256184,-0.317195968905306,
0.962485392528369));
#19916=CARTESIAN_POINT('Ctrl Pts',(1.36127834356734,-0.266264900654909,
0.920778333482565));
#19917=CARTESIAN_POINT('Ctrl Pts',(1.3735491215176,-0.237231147975234,0.902193646979983));
#19918=CARTESIAN_POINT('Ctrl Pts',(1.39550172959303,-0.166543350814306,
0.867957148219442));
#19919=CARTESIAN_POINT('Ctrl Pts',(1.40380622184538,-0.123401821157026,
0.854205272175555));
#19920=CARTESIAN_POINT('Ctrl Pts',(1.40825612658882,-0.0793800000000001,
0.846804978391753));
#19921=CARTESIAN_POINT('',(0.886256117232623,-0.07938,1.45861320581289));
#19922=CARTESIAN_POINT('Origin',(1.18440385848747,-0.07938,1.18440385848747));
#19923=CARTESIAN_POINT('',(1.45861320581289,-0.07938,0.886256117232624));
#19924=CARTESIAN_POINT('Ctrl Pts',(1.45861320581289,-0.0793800000000001,
0.886256117232623));
#19925=CARTESIAN_POINT('Ctrl Pts',(1.45630208793976,-0.101649918886749,
0.890059788636852));
#19926=CARTESIAN_POINT('Ctrl Pts',(1.45296717977858,-0.123823518623746,
0.895520212222107));
#19927=CARTESIAN_POINT('Ctrl Pts',(1.43904931717599,-0.192480977588836,
0.917859913453975));
#19928=CARTESIAN_POINT('Ctrl Pts',(1.4243271592157,-0.236152929235938,0.940896403863072));
#19929=CARTESIAN_POINT('Ctrl Pts',(1.39055359345152,-0.303141259068212,
0.990027513266106));
#19930=CARTESIAN_POINT('Ctrl Pts',(1.36743459453896,-0.335108247315849,
1.02199477007745));
#19931=CARTESIAN_POINT('Ctrl Pts',(1.32643091652006,-0.373243761060364,
1.07446535104584));
#19932=CARTESIAN_POINT('Ctrl Pts',(1.30441816675528,-0.387888272594439,
1.10126842659597));
#19933=CARTESIAN_POINT('Ctrl Pts',(1.25681160160691,-0.407041111792943,
1.15530234155453));
#19934=CARTESIAN_POINT('Ctrl Pts',(1.23119764287622,-0.411552957311693,
1.18251418313119));
#19935=CARTESIAN_POINT('Ctrl Pts',(1.18251418313119,-0.411552957311693,
1.23119764287622));
#19936=CARTESIAN_POINT('Ctrl Pts',(1.15530234155453,-0.407041111792943,
1.25681160160691));
#19937=CARTESIAN_POINT('Ctrl Pts',(1.10126842659597,-0.387888272594439,
1.30441816675528));
#19938=CARTESIAN_POINT('Ctrl Pts',(1.07446535104584,-0.373243761060364,
1.32643091652006));
#19939=CARTESIAN_POINT('Ctrl Pts',(1.02199477007745,-0.335108247315848,
1.36743459453896));
#19940=CARTESIAN_POINT('Ctrl Pts',(0.990027513266105,-0.303141259068211,
1.39055359345152));
#19941=CARTESIAN_POINT('Ctrl Pts',(0.940896403863071,-0.236152929235937,
1.42432715921571));
#19942=CARTESIAN_POINT('Ctrl Pts',(0.917859913453974,-0.192480977588835,
1.43904931717599));
#19943=CARTESIAN_POINT('Ctrl Pts',(0.895520212222106,-0.123823518623745,
1.45296717977858));
#19944=CARTESIAN_POINT('Ctrl Pts',(0.890059788636851,-0.101649918886749,
1.45630208793976));
#19945=CARTESIAN_POINT('Ctrl Pts',(0.886256117232622,-0.0793800000000001,
1.45861320581289));
#19946=CARTESIAN_POINT('Origin',(1.18440385848747,-0.07938,1.18440385848747));
#19947=CARTESIAN_POINT('Origin',(0.,-0.27783,0.));
#19948=CARTESIAN_POINT('',(0.404717578595295,-0.07938,1.65807299932179));
#19949=CARTESIAN_POINT('Origin',(0.,-0.07938,0.));
#19950=CARTESIAN_POINT('',(-0.404717578595296,-0.07938,1.65807299932179));
#19951=CARTESIAN_POINT('Ctrl Pts',(0.404717578595296,-0.0793800000000001,
1.65807299932179));
#19952=CARTESIAN_POINT('Ctrl Pts',(0.400393769631747,-0.101649918886749,
1.65912839404491));
#19953=CARTESIAN_POINT('Ctrl Pts',(0.394174530911058,-0.123823518623745,
1.66063136041479));
#19954=CARTESIAN_POINT('Ctrl Pts',(0.368536561654407,-0.192480977588835,
1.66658649961961));
#19955=CARTESIAN_POINT('Ctrl Pts',(0.341837165343982,-0.236152929235937,
1.67246562047521));
#19956=CARTESIAN_POINT('Ctrl Pts',(0.283214707341173,-0.303141259068211,
1.68332504372461));
#19957=CARTESIAN_POINT('Ctrl Pts',(0.244262842368623,-0.335108247315849,
1.68958170688653));
#19958=CARTESIAN_POINT('Ctrl Pts',(0.178166559972324,-0.373243761060364,
1.69769003172132));
#19959=CARTESIAN_POINT('Ctrl Pts',(0.143648558862931,-0.387888272594439,
1.70107730356824));
#19960=CARTESIAN_POINT('Ctrl Pts',(0.0717778861362652,-0.407041111792943,
1.70562212620408));
#19961=CARTESIAN_POINT('Ctrl Pts',(0.0344244045173309,-0.411552957311693,
1.706752));
#19962=CARTESIAN_POINT('Ctrl Pts',(-0.0344244045173315,-0.411552957311693,
1.706752));
#19963=CARTESIAN_POINT('Ctrl Pts',(-0.0717778861362658,-0.407041111792943,
1.70562212620408));
#19964=CARTESIAN_POINT('Ctrl Pts',(-0.143648558862932,-0.387888272594439,
1.70107730356824));
#19965=CARTESIAN_POINT('Ctrl Pts',(-0.178166559972325,-0.373243761060364,
1.69769003172132));
#19966=CARTESIAN_POINT('Ctrl Pts',(-0.244262842368624,-0.335108247315849,
1.68958170688653));
#19967=CARTESIAN_POINT('Ctrl Pts',(-0.283214707341173,-0.303141259068212,
1.68332504372461));
#19968=CARTESIAN_POINT('Ctrl Pts',(-0.341837165343982,-0.236152929235937,
1.67246562047521));
#19969=CARTESIAN_POINT('Ctrl Pts',(-0.368536561654408,-0.192480977588835,
1.66658649961961));
#19970=CARTESIAN_POINT('Ctrl Pts',(-0.394174530911059,-0.123823518623745,
1.66063136041479));
#19971=CARTESIAN_POINT('Ctrl Pts',(-0.400393769631748,-0.101649918886749,
1.65912839404491));
#19972=CARTESIAN_POINT('Ctrl Pts',(-0.404717578595297,-0.0793800000000001,
1.65807299932179));
#19973=CARTESIAN_POINT('',(-0.886256117232624,-0.07938,1.45861320581289));
#19974=CARTESIAN_POINT('Origin',(0.,-0.07938,0.));
#19975=CARTESIAN_POINT('',(-1.45861320581289,-0.07938,0.886256117232623));
#19976=CARTESIAN_POINT('Ctrl Pts',(-0.886256117232623,-0.0793800000000001,
1.45861320581289));
#19977=CARTESIAN_POINT('Ctrl Pts',(-0.890059788636852,-0.101649918886749,
1.45630208793976));
#19978=CARTESIAN_POINT('Ctrl Pts',(-0.895520212222106,-0.123823518623745,
1.45296717977858));
#19979=CARTESIAN_POINT('Ctrl Pts',(-0.917859913453974,-0.192480977588835,
1.43904931717599));
#19980=CARTESIAN_POINT('Ctrl Pts',(-0.940896403863071,-0.236152929235937,
1.4243271592157));
#19981=CARTESIAN_POINT('Ctrl Pts',(-0.990027513266105,-0.303141259068211,
1.39055359345152));
#19982=CARTESIAN_POINT('Ctrl Pts',(-1.02199477007745,-0.335108247315848,
1.36743459453896));
#19983=CARTESIAN_POINT('Ctrl Pts',(-1.07446535104584,-0.373243761060364,
1.32643091652006));
#19984=CARTESIAN_POINT('Ctrl Pts',(-1.10126842659597,-0.387888272594439,
1.30441816675528));
#19985=CARTESIAN_POINT('Ctrl Pts',(-1.15530234155453,-0.407041111792943,
1.25681160160691));
#19986=CARTESIAN_POINT('Ctrl Pts',(-1.18251418313119,-0.411552957311693,
1.23119764287622));
#19987=CARTESIAN_POINT('Ctrl Pts',(-1.23119764287622,-0.411552957311693,
1.18251418313119));
#19988=CARTESIAN_POINT('Ctrl Pts',(-1.25681160160691,-0.407041111792943,
1.15530234155453));
#19989=CARTESIAN_POINT('Ctrl Pts',(-1.30441816675528,-0.387888272594439,
1.10126842659597));
#19990=CARTESIAN_POINT('Ctrl Pts',(-1.32643091652006,-0.373243761060365,
1.07446535104584));
#19991=CARTESIAN_POINT('Ctrl Pts',(-1.36743459453896,-0.335108247315849,
1.02199477007745));
#19992=CARTESIAN_POINT('Ctrl Pts',(-1.39055359345152,-0.303141259068212,
0.990027513266106));
#19993=CARTESIAN_POINT('Ctrl Pts',(-1.4243271592157,-0.236152929235938,
0.940896403863071));
#19994=CARTESIAN_POINT('Ctrl Pts',(-1.43904931717599,-0.192480977588836,
0.917859913453974));
#19995=CARTESIAN_POINT('Ctrl Pts',(-1.45296717977858,-0.123823518623746,
0.895520212222106));
#19996=CARTESIAN_POINT('Ctrl Pts',(-1.45630208793976,-0.101649918886749,
0.890059788636852));
#19997=CARTESIAN_POINT('Ctrl Pts',(-1.45861320581289,-0.0793800000000001,
0.886256117232623));
#19998=CARTESIAN_POINT('',(-1.65807299932179,-0.07938,0.404717578595295));
#19999=CARTESIAN_POINT('Origin',(0.,-0.07938,0.));
#20000=CARTESIAN_POINT('',(-1.706752,-0.411552957311693,2.08591827245526E-16));
#20001=CARTESIAN_POINT('Ctrl Pts',(-1.65807299932179,-0.0793800000000001,
0.404717578595296));
#20002=CARTESIAN_POINT('Ctrl Pts',(-1.65912839404491,-0.101649918886749,
0.400393769631747));
#20003=CARTESIAN_POINT('Ctrl Pts',(-1.66063136041479,-0.123823518623745,
0.394174530911058));
#20004=CARTESIAN_POINT('Ctrl Pts',(-1.66658649961961,-0.192480977588835,
0.368536561654407));
#20005=CARTESIAN_POINT('Ctrl Pts',(-1.67246562047521,-0.236152929235937,
0.341837165343982));
#20006=CARTESIAN_POINT('Ctrl Pts',(-1.68332504372461,-0.303141259068211,
0.283214707341173));
#20007=CARTESIAN_POINT('Ctrl Pts',(-1.68958170688653,-0.335108247315848,
0.244262842368623));
#20008=CARTESIAN_POINT('Ctrl Pts',(-1.69769003172132,-0.373243761060364,
0.178166559972324));
#20009=CARTESIAN_POINT('Ctrl Pts',(-1.70107730356824,-0.387888272594439,
0.143648558862931));
#20010=CARTESIAN_POINT('Ctrl Pts',(-1.70562212620408,-0.407041111792943,
0.0717778861362656));
#20011=CARTESIAN_POINT('Ctrl Pts',(-1.706752,-0.411552957311693,0.0344244045173313));
#20012=CARTESIAN_POINT('Ctrl Pts',(-1.706752,-0.411552957311693,2.08166817117217E-16));
#20013=CARTESIAN_POINT('',(-1.706752,-0.47628,2.09016837373834E-16));
#20014=CARTESIAN_POINT('',(-1.706752,-0.27783,2.09016837373834E-16));
#20015=CARTESIAN_POINT('Origin',(0.,-0.47628,0.));
#20016=CARTESIAN_POINT('',(-1.65807299932179,-0.07938,-0.404717578595296));
#20017=CARTESIAN_POINT('Ctrl Pts',(-1.706752,-0.411552957311693,2.0122792321331E-16));
#20018=CARTESIAN_POINT('Ctrl Pts',(-1.706752,-0.411552957311693,-0.0344244045173309));
#20019=CARTESIAN_POINT('Ctrl Pts',(-1.70562212620408,-0.407041111792943,
-0.0717778861362652));
#20020=CARTESIAN_POINT('Ctrl Pts',(-1.70107730356824,-0.387888272594439,
-0.143648558862931));
#20021=CARTESIAN_POINT('Ctrl Pts',(-1.69769003172132,-0.373243761060365,
-0.178166559972324));
#20022=CARTESIAN_POINT('Ctrl Pts',(-1.68958170688653,-0.335108247315849,
-0.244262842368623));
#20023=CARTESIAN_POINT('Ctrl Pts',(-1.68332504372461,-0.303141259068212,
-0.283214707341173));
#20024=CARTESIAN_POINT('Ctrl Pts',(-1.67246562047521,-0.236152929235938,
-0.341837165343982));
#20025=CARTESIAN_POINT('Ctrl Pts',(-1.66658649961961,-0.192480977588836,
-0.368536561654407));
#20026=CARTESIAN_POINT('Ctrl Pts',(-1.66063136041479,-0.123823518623745,
-0.394174530911059));
#20027=CARTESIAN_POINT('Ctrl Pts',(-1.65912839404491,-0.101649918886749,
-0.400393769631748));
#20028=CARTESIAN_POINT('Ctrl Pts',(-1.65807299932179,-0.0793800000000001,
-0.404717578595296));
#20029=CARTESIAN_POINT('',(-1.45861320581289,-0.07938,-0.886256117232623));
#20030=CARTESIAN_POINT('Origin',(0.,-0.07938,0.));
#20031=CARTESIAN_POINT('',(-0.886256117232623,-0.07938,-1.45861320581289));
#20032=CARTESIAN_POINT('Ctrl Pts',(-1.45861320581289,-0.0793800000000001,
-0.886256117232623));
#20033=CARTESIAN_POINT('Ctrl Pts',(-1.45630208793976,-0.101649918886749,
-0.890059788636852));
#20034=CARTESIAN_POINT('Ctrl Pts',(-1.45296717977858,-0.123823518623745,
-0.895520212222106));
#20035=CARTESIAN_POINT('Ctrl Pts',(-1.43904931717599,-0.192480977588835,
-0.917859913453974));
#20036=CARTESIAN_POINT('Ctrl Pts',(-1.4243271592157,-0.236152929235937,
-0.940896403863072));
#20037=CARTESIAN_POINT('Ctrl Pts',(-1.39055359345152,-0.303141259068212,
-0.990027513266106));
#20038=CARTESIAN_POINT('Ctrl Pts',(-1.36743459453896,-0.335108247315849,
-1.02199477007745));
#20039=CARTESIAN_POINT('Ctrl Pts',(-1.32643091652006,-0.373243761060364,
-1.07446535104584));
#20040=CARTESIAN_POINT('Ctrl Pts',(-1.30441816675528,-0.387888272594439,
-1.10126842659597));
#20041=CARTESIAN_POINT('Ctrl Pts',(-1.25681160160691,-0.407041111792943,
-1.15530234155453));
#20042=CARTESIAN_POINT('Ctrl Pts',(-1.23119764287622,-0.411552957311693,
-1.18251418313119));
#20043=CARTESIAN_POINT('Ctrl Pts',(-1.18251418313119,-0.411552957311693,
-1.23119764287622));
#20044=CARTESIAN_POINT('Ctrl Pts',(-1.15530234155453,-0.407041111792943,
-1.25681160160691));
#20045=CARTESIAN_POINT('Ctrl Pts',(-1.10126842659597,-0.387888272594439,
-1.30441816675528));
#20046=CARTESIAN_POINT('Ctrl Pts',(-1.07446535104584,-0.373243761060364,
-1.32643091652006));
#20047=CARTESIAN_POINT('Ctrl Pts',(-1.02199477007745,-0.335108247315848,
-1.36743459453896));
#20048=CARTESIAN_POINT('Ctrl Pts',(-0.990027513266105,-0.303141259068211,
-1.39055359345152));
#20049=CARTESIAN_POINT('Ctrl Pts',(-0.940896403863071,-0.236152929235936,
-1.42432715921571));
#20050=CARTESIAN_POINT('Ctrl Pts',(-0.917859913453974,-0.192480977588835,
-1.43904931717599));
#20051=CARTESIAN_POINT('Ctrl Pts',(-0.895520212222106,-0.123823518623745,
-1.45296717977858));
#20052=CARTESIAN_POINT('Ctrl Pts',(-0.890059788636851,-0.101649918886749,
-1.45630208793976));
#20053=CARTESIAN_POINT('Ctrl Pts',(-0.886256117232623,-0.0793800000000001,
-1.45861320581289));
#20054=CARTESIAN_POINT('',(-0.404717578595295,-0.07938,-1.65807299932179));
#20055=CARTESIAN_POINT('Origin',(0.,-0.07938,0.));
#20056=CARTESIAN_POINT('',(0.404717578595296,-0.07938,-1.65807299932179));
#20057=CARTESIAN_POINT('Ctrl Pts',(-0.404717578595296,-0.0793800000000001,
-1.65807299932179));
#20058=CARTESIAN_POINT('Ctrl Pts',(-0.400393769631747,-0.101649918886749,
-1.65912839404491));
#20059=CARTESIAN_POINT('Ctrl Pts',(-0.394174530911058,-0.123823518623746,
-1.66063136041479));
#20060=CARTESIAN_POINT('Ctrl Pts',(-0.368536561654407,-0.192480977588836,
-1.66658649961961));
#20061=CARTESIAN_POINT('Ctrl Pts',(-0.341837165343982,-0.236152929235938,
-1.67246562047521));
#20062=CARTESIAN_POINT('Ctrl Pts',(-0.283214707341173,-0.303141259068212,
-1.68332504372461));
#20063=CARTESIAN_POINT('Ctrl Pts',(-0.244262842368623,-0.335108247315849,
-1.68958170688653));
#20064=CARTESIAN_POINT('Ctrl Pts',(-0.178166559972324,-0.373243761060364,
-1.69769003172132));
#20065=CARTESIAN_POINT('Ctrl Pts',(-0.143648558862931,-0.387888272594439,
-1.70107730356824));
#20066=CARTESIAN_POINT('Ctrl Pts',(-0.0717778861362653,-0.407041111792943,
-1.70562212620408));
#20067=CARTESIAN_POINT('Ctrl Pts',(-0.034424404517331,-0.411552957311693,
-1.706752));
#20068=CARTESIAN_POINT('Ctrl Pts',(0.0344244045173312,-0.411552957311693,
-1.706752));
#20069=CARTESIAN_POINT('Ctrl Pts',(0.0717778861362655,-0.407041111792943,
-1.70562212620408));
#20070=CARTESIAN_POINT('Ctrl Pts',(0.143648558862931,-0.387888272594439,
-1.70107730356824));
#20071=CARTESIAN_POINT('Ctrl Pts',(0.178166559972324,-0.373243761060364,
-1.69769003172132));
#20072=CARTESIAN_POINT('Ctrl Pts',(0.244262842368623,-0.335108247315849,
-1.68958170688653));
#20073=CARTESIAN_POINT('Ctrl Pts',(0.283214707341173,-0.303141259068212,
-1.68332504372461));
#20074=CARTESIAN_POINT('Ctrl Pts',(0.341837165343982,-0.236152929235937,
-1.67246562047521));
#20075=CARTESIAN_POINT('Ctrl Pts',(0.368536561654407,-0.192480977588835,
-1.66658649961961));
#20076=CARTESIAN_POINT('Ctrl Pts',(0.394174530911059,-0.123823518623745,
-1.66063136041479));
#20077=CARTESIAN_POINT('Ctrl Pts',(0.400393769631748,-0.101649918886749,
-1.65912839404491));
#20078=CARTESIAN_POINT('Ctrl Pts',(0.404717578595296,-0.0793800000000001,
-1.65807299932179));
#20079=CARTESIAN_POINT('',(0.886256117232623,-0.07938,-1.45861320581289));
#20080=CARTESIAN_POINT('Origin',(0.,-0.07938,0.));
#20081=CARTESIAN_POINT('',(1.45861320581289,-0.07938,-0.886256117232623));
#20082=CARTESIAN_POINT('Ctrl Pts',(0.886256117232623,-0.0793800000000001,
-1.45861320581289));
#20083=CARTESIAN_POINT('Ctrl Pts',(0.890059788636852,-0.101649918886749,
-1.45630208793976));
#20084=CARTESIAN_POINT('Ctrl Pts',(0.895520212222106,-0.123823518623745,
-1.45296717977858));
#20085=CARTESIAN_POINT('Ctrl Pts',(0.917859913453974,-0.192480977588835,
-1.43904931717599));
#20086=CARTESIAN_POINT('Ctrl Pts',(0.940896403863072,-0.236152929235937,
-1.4243271592157));
#20087=CARTESIAN_POINT('Ctrl Pts',(0.990027513266106,-0.303141259068211,
-1.39055359345152));
#20088=CARTESIAN_POINT('Ctrl Pts',(1.02199477007745,-0.335108247315849,
-1.36743459453896));
#20089=CARTESIAN_POINT('Ctrl Pts',(1.07446535104584,-0.373243761060364,
-1.32643091652006));
#20090=CARTESIAN_POINT('Ctrl Pts',(1.10126842659597,-0.387888272594439,
-1.30441816675528));
#20091=CARTESIAN_POINT('Ctrl Pts',(1.15530234155453,-0.407041111792943,
-1.25681160160691));
#20092=CARTESIAN_POINT('Ctrl Pts',(1.18251418313119,-0.411552957311693,
-1.23119764287622));
#20093=CARTESIAN_POINT('Ctrl Pts',(1.23119764287622,-0.411552957311693,
-1.18251418313119));
#20094=CARTESIAN_POINT('Ctrl Pts',(1.25681160160691,-0.407041111792943,
-1.15530234155453));
#20095=CARTESIAN_POINT('Ctrl Pts',(1.30441816675528,-0.387888272594439,
-1.10126842659597));
#20096=CARTESIAN_POINT('Ctrl Pts',(1.32643091652006,-0.373243761060364,
-1.07446535104584));
#20097=CARTESIAN_POINT('Ctrl Pts',(1.36743459453896,-0.335108247315849,
-1.02199477007745));
#20098=CARTESIAN_POINT('Ctrl Pts',(1.39055359345152,-0.303141259068212,
-0.990027513266105));
#20099=CARTESIAN_POINT('Ctrl Pts',(1.4243271592157,-0.236152929235937,-0.940896403863071));
#20100=CARTESIAN_POINT('Ctrl Pts',(1.43904931717599,-0.192480977588835,
-0.917859913453974));
#20101=CARTESIAN_POINT('Ctrl Pts',(1.45296717977858,-0.123823518623745,
-0.895520212222106));
#20102=CARTESIAN_POINT('Ctrl Pts',(1.45630208793976,-0.101649918886749,
-0.890059788636852));
#20103=CARTESIAN_POINT('Ctrl Pts',(1.45861320581289,-0.0793800000000001,
-0.886256117232623));
#20104=CARTESIAN_POINT('',(1.65807299932179,-0.07938,-0.404717578595296));
#20105=CARTESIAN_POINT('Origin',(0.,-0.07938,0.));
#20106=CARTESIAN_POINT('',(1.65807299932179,-0.07938,0.404717578595296));
#20107=CARTESIAN_POINT('Ctrl Pts',(1.65807299932179,-0.0793800000000001,
-0.404717578595296));
#20108=CARTESIAN_POINT('Ctrl Pts',(1.65912839404491,-0.101649918886749,
-0.400393769631747));
#20109=CARTESIAN_POINT('Ctrl Pts',(1.66063136041479,-0.123823518623745,
-0.394174530911058));
#20110=CARTESIAN_POINT('Ctrl Pts',(1.66658649961961,-0.192480977588835,
-0.368536561654407));
#20111=CARTESIAN_POINT('Ctrl Pts',(1.67246562047521,-0.236152929235937,
-0.341837165343982));
#20112=CARTESIAN_POINT('Ctrl Pts',(1.68332504372461,-0.303141259068212,
-0.283214707341173));
#20113=CARTESIAN_POINT('Ctrl Pts',(1.68958170688653,-0.335108247315849,
-0.244262842368623));
#20114=CARTESIAN_POINT('Ctrl Pts',(1.69769003172132,-0.373243761060364,
-0.178166559972324));
#20115=CARTESIAN_POINT('Ctrl Pts',(1.70107730356824,-0.387888272594439,
-0.143648558862931));
#20116=CARTESIAN_POINT('Ctrl Pts',(1.70562212620408,-0.407041111792943,
-0.0717778861362655));
#20117=CARTESIAN_POINT('Ctrl Pts',(1.706752,-0.411552957311693,-0.0344244045173312));
#20118=CARTESIAN_POINT('Ctrl Pts',(1.706752,-0.411552957311693,0.0344244045173312));
#20119=CARTESIAN_POINT('Ctrl Pts',(1.70562212620408,-0.407041111792943,
0.0717778861362655));
#20120=CARTESIAN_POINT('Ctrl Pts',(1.70107730356824,-0.387888272594439,
0.143648558862931));
#20121=CARTESIAN_POINT('Ctrl Pts',(1.69769003172132,-0.373243761060364,
0.178166559972324));
#20122=CARTESIAN_POINT('Ctrl Pts',(1.68958170688653,-0.335108247315849,
0.244262842368623));
#20123=CARTESIAN_POINT('Ctrl Pts',(1.68332504372461,-0.303141259068212,
0.283214707341173));
#20124=CARTESIAN_POINT('Ctrl Pts',(1.67246562047521,-0.236152929235937,
0.341837165343982));
#20125=CARTESIAN_POINT('Ctrl Pts',(1.66658649961961,-0.192480977588835,
0.368536561654407));
#20126=CARTESIAN_POINT('Ctrl Pts',(1.66063136041479,-0.123823518623745,
0.394174530911058));
#20127=CARTESIAN_POINT('Ctrl Pts',(1.65912839404491,-0.101649918886749,
0.400393769631747));
#20128=CARTESIAN_POINT('Ctrl Pts',(1.65807299932179,-0.0793800000000001,
0.404717578595296));
#20129=CARTESIAN_POINT('Origin',(0.,-0.07938,0.));
#20130=CARTESIAN_POINT('Origin',(0.,-0.07938,0.));
#20131=CARTESIAN_POINT('',(0.397005914195118,-0.07938,1.59456899932179));
#20132=CARTESIAN_POINT('Origin',(0.,-0.07938,0.));
#20133=CARTESIAN_POINT('Origin',(-3.33066907387547E-16,-0.07938,1.675));
#20134=CARTESIAN_POINT('Origin',(-3.33066907387547E-16,0.,1.675));
#20135=CARTESIAN_POINT('',(-0.397005914195118,-0.07938,1.59456899932179));
#20136=CARTESIAN_POINT('Ctrl Pts',(-0.397005914195119,-0.0793800000000001,
1.59456899932179));
#20137=CARTESIAN_POINT('Ctrl Pts',(-0.3886265584581,-0.123401821157026,
1.59665523941937));
#20138=CARTESIAN_POINT('Ctrl Pts',(-0.373030350867485,-0.166543350814306,
1.60050712143809));
#20139=CARTESIAN_POINT('Ctrl Pts',(-0.333298652394954,-0.237231147975234,
1.60919314384089));
#20140=CARTESIAN_POINT('Ctrl Pts',(-0.311480544243687,-0.266264900654909,
1.61365775139403));
#20141=CARTESIAN_POINT('Ctrl Pts',(-0.261368388670537,-0.317195968905306,
1.62252828437015));
#20142=CARTESIAN_POINT('Ctrl Pts',(-0.233069203882014,-0.33909093068465,
1.62691869420078));
#20143=CARTESIAN_POINT('Ctrl Pts',(-0.174042761838764,-0.373586846396559,
1.63426473152765));
#20144=CARTESIAN_POINT('Ctrl Pts',(-0.14036578147155,-0.388086240756494,
1.63761964365402));
#20145=CARTESIAN_POINT('Ctrl Pts',(-0.0701778381840615,-0.407068917407805,
1.64212536811722));
#20146=CARTESIAN_POINT('Ctrl Pts',(-0.0336652739555918,-0.411552957311693,
1.643248));
#20147=CARTESIAN_POINT('Ctrl Pts',(0.0336652739555913,-0.411552957311693,
1.643248));
#20148=CARTESIAN_POINT('Ctrl Pts',(0.070177838184061,-0.407068917407805,
1.64212536811722));
#20149=CARTESIAN_POINT('Ctrl Pts',(0.140365781471549,-0.388086240756494,
1.63761964365402));
#20150=CARTESIAN_POINT('Ctrl Pts',(0.174042761838763,-0.373586846396559,
1.63426473152765));
#20151=CARTESIAN_POINT('Ctrl Pts',(0.233069203882014,-0.33909093068465,
1.62691869420078));
#20152=CARTESIAN_POINT('Ctrl Pts',(0.261368388670536,-0.317195968905306,
1.62252828437015));
#20153=CARTESIAN_POINT('Ctrl Pts',(0.311480544243686,-0.266264900654908,
1.61365775139403));
#20154=CARTESIAN_POINT('Ctrl Pts',(0.333298652394954,-0.237231147975234,
1.60919314384089));
#20155=CARTESIAN_POINT('Ctrl Pts',(0.373030350867484,-0.166543350814306,
1.60050712143809));
#20156=CARTESIAN_POINT('Ctrl Pts',(0.388626558458099,-0.123401821157026,
1.59665523941937));
#20157=CARTESIAN_POINT('Ctrl Pts',(0.397005914195118,-0.07938,1.59456899932179));
#20158=CARTESIAN_POINT('Origin',(-3.33066907387547E-16,-0.07938,1.675));
#20159=CARTESIAN_POINT('Origin',(0.,-0.07938,0.));
#20160=CARTESIAN_POINT('',(-0.846804978391754,-0.07938,1.40825612658882));
#20161=CARTESIAN_POINT('Origin',(0.,-0.07938,0.));
#20162=CARTESIAN_POINT('Origin',(-1.18440385848747,-0.07938,1.18440385848747));
#20163=CARTESIAN_POINT('Origin',(-1.18440385848747,0.,1.18440385848747));
#20164=CARTESIAN_POINT('',(-1.40825612658882,-0.07938,0.846804978391753));
#20165=CARTESIAN_POINT('Ctrl Pts',(-1.40825612658882,-0.0793800000000001,
0.846804978391753));
#20166=CARTESIAN_POINT('Ctrl Pts',(-1.40380622184538,-0.123401821157026,
0.854205272175555));
#20167=CARTESIAN_POINT('Ctrl Pts',(-1.39550172959303,-0.166543350814306,
0.867957148219442));
#20168=CARTESIAN_POINT('Ctrl Pts',(-1.3735491215176,-0.237231147975235,
0.902193646979983));
#20169=CARTESIAN_POINT('Ctrl Pts',(-1.36127834356734,-0.266264900654909,
0.920778333482565));
#20170=CARTESIAN_POINT('Ctrl Pts',(-1.33211611256184,-0.317195968905306,
0.962485392528369));
#20171=CARTESIAN_POINT('Ctrl Pts',(-1.31521005565926,-0.339090930684651,
0.985600426557816));
#20172=CARTESIAN_POINT('Ctrl Pts',(-1.27866649102984,-0.373586846396559,
1.03253285680459));
#20173=CARTESIAN_POINT('Ctrl Pts',(-1.25722555095714,-0.388086240756494,
1.05871835910697));
#20174=CARTESIAN_POINT('Ctrl Pts',(-1.2107812086231,-0.407068917407805,
1.11153475808518));
#20175=CARTESIAN_POINT('Ctrl Pts',(-1.18575674747573,-0.411552957311693,
1.13814686046673));
#20176=CARTESIAN_POINT('Ctrl Pts',(-1.13814686046673,-0.411552957311693,
1.18575674747573));
#20177=CARTESIAN_POINT('Ctrl Pts',(-1.11153475808518,-0.407068917407805,
1.2107812086231));
#20178=CARTESIAN_POINT('Ctrl Pts',(-1.05871835910697,-0.388086240756494,
1.25722555095714));
#20179=CARTESIAN_POINT('Ctrl Pts',(-1.03253285680459,-0.373586846396559,
1.27866649102984));
#20180=CARTESIAN_POINT('Ctrl Pts',(-0.985600426557816,-0.33909093068465,
1.31521005565926));
#20181=CARTESIAN_POINT('Ctrl Pts',(-0.962485392528369,-0.317195968905306,
1.33211611256184));
#20182=CARTESIAN_POINT('Ctrl Pts',(-0.920778333482565,-0.266264900654908,
1.36127834356734));
#20183=CARTESIAN_POINT('Ctrl Pts',(-0.902193646979983,-0.237231147975234,
1.3735491215176));
#20184=CARTESIAN_POINT('Ctrl Pts',(-0.867957148219442,-0.166543350814306,
1.39550172959303));
#20185=CARTESIAN_POINT('Ctrl Pts',(-0.854205272175555,-0.123401821157026,
1.40380622184538));
#20186=CARTESIAN_POINT('Ctrl Pts',(-0.846804978391753,-0.0793800000000001,
1.40825612658882));
#20187=CARTESIAN_POINT('Origin',(-1.18440385848747,-0.07938,1.18440385848747));
#20188=CARTESIAN_POINT('Origin',(0.,-0.07938,0.));
#20189=CARTESIAN_POINT('',(-1.59456899932179,-0.07938,0.397005914195118));
#20190=CARTESIAN_POINT('Origin',(0.,-0.07938,0.));
#20191=CARTESIAN_POINT('Origin',(-1.675,-0.07938,-2.22044604925031E-16));
#20192=CARTESIAN_POINT('Origin',(-1.675,0.,-2.22044604925031E-16));
#20193=CARTESIAN_POINT('',(-1.59456899932179,-0.07938,-0.397005914195118));
#20194=CARTESIAN_POINT('',(-1.643248,-0.411552957311693,3.47540551556327E-18));
#20195=CARTESIAN_POINT('Ctrl Pts',(-1.59456899932179,-0.0793800000000001,
-0.397005914195119));
#20196=CARTESIAN_POINT('Ctrl Pts',(-1.59665523941937,-0.123401821157026,
-0.388626558458099));
#20197=CARTESIAN_POINT('Ctrl Pts',(-1.60050712143809,-0.166543350814306,
-0.373030350867485));
#20198=CARTESIAN_POINT('Ctrl Pts',(-1.60919314384089,-0.237231147975234,
-0.333298652394954));
#20199=CARTESIAN_POINT('Ctrl Pts',(-1.61365775139403,-0.266264900654909,
-0.311480544243686));
#20200=CARTESIAN_POINT('Ctrl Pts',(-1.62252828437015,-0.317195968905306,
-0.261368388670537));
#20201=CARTESIAN_POINT('Ctrl Pts',(-1.62691869420078,-0.33909093068465,
-0.233069203882014));
#20202=CARTESIAN_POINT('Ctrl Pts',(-1.63426473152765,-0.373586846396559,
-0.174042761838764));
#20203=CARTESIAN_POINT('Ctrl Pts',(-1.63761964365402,-0.388086240756494,
-0.140365781471549));
#20204=CARTESIAN_POINT('Ctrl Pts',(-1.64212536811722,-0.407068917407805,
-0.0701778381840614));
#20205=CARTESIAN_POINT('Ctrl Pts',(-1.643248,-0.411552957311693,-0.0336652739555917));
#20206=CARTESIAN_POINT('Ctrl Pts',(-1.643248,-0.411552957311693,-2.0122792321331E-16));
#20207=CARTESIAN_POINT('Origin',(-1.675,-0.07938,-2.22044604925031E-16));
#20208=CARTESIAN_POINT('Ctrl Pts',(-1.643248,-0.411552957311693,-1.94289029309402E-16));
#20209=CARTESIAN_POINT('Ctrl Pts',(-1.643248,-0.411552957311693,0.0336652739555913));
#20210=CARTESIAN_POINT('Ctrl Pts',(-1.64212536811722,-0.407068917407805,
0.0701778381840609));
#20211=CARTESIAN_POINT('Ctrl Pts',(-1.63761964365402,-0.388086240756494,
0.140365781471549));
#20212=CARTESIAN_POINT('Ctrl Pts',(-1.63426473152765,-0.373586846396559,
0.174042761838763));
#20213=CARTESIAN_POINT('Ctrl Pts',(-1.62691869420078,-0.33909093068465,
0.233069203882014));
#20214=CARTESIAN_POINT('Ctrl Pts',(-1.62252828437015,-0.317195968905306,
0.261368388670536));
#20215=CARTESIAN_POINT('Ctrl Pts',(-1.61365775139403,-0.266264900654909,
0.311480544243686));
#20216=CARTESIAN_POINT('Ctrl Pts',(-1.60919314384089,-0.237231147975235,
0.333298652394954));
#20217=CARTESIAN_POINT('Ctrl Pts',(-1.60050712143809,-0.166543350814306,
0.373030350867484));
#20218=CARTESIAN_POINT('Ctrl Pts',(-1.59665523941937,-0.123401821157026,
0.388626558458099));
#20219=CARTESIAN_POINT('Ctrl Pts',(-1.59456899932179,-0.0793800000000001,
0.397005914195118));
#20220=CARTESIAN_POINT('Origin',(0.,-0.07938,0.));
#20221=CARTESIAN_POINT('',(-1.40825612658882,-0.07938,-0.846804978391753));
#20222=CARTESIAN_POINT('Origin',(0.,-0.07938,0.));
#20223=CARTESIAN_POINT('Origin',(-1.18440385848747,-0.07938,-1.18440385848747));
#20224=CARTESIAN_POINT('Origin',(-1.18440385848747,0.,-1.18440385848747));
#20225=CARTESIAN_POINT('',(-0.846804978391753,-0.07938,-1.40825612658882));
#20226=CARTESIAN_POINT('Ctrl Pts',(-0.846804978391753,-0.0793800000000001,
-1.40825612658882));
#20227=CARTESIAN_POINT('Ctrl Pts',(-0.854205272175555,-0.123401821157026,
-1.40380622184538));
#20228=CARTESIAN_POINT('Ctrl Pts',(-0.867957148219442,-0.166543350814306,
-1.39550172959303));
#20229=CARTESIAN_POINT('Ctrl Pts',(-0.902193646979982,-0.237231147975234,
-1.3735491215176));
#20230=CARTESIAN_POINT('Ctrl Pts',(-0.920778333482564,-0.266264900654908,
-1.36127834356734));
#20231=CARTESIAN_POINT('Ctrl Pts',(-0.962485392528368,-0.317195968905306,
-1.33211611256184));
#20232=CARTESIAN_POINT('Ctrl Pts',(-0.985600426557816,-0.33909093068465,
-1.31521005565926));
#20233=CARTESIAN_POINT('Ctrl Pts',(-1.03253285680459,-0.373586846396559,
-1.27866649102984));
#20234=CARTESIAN_POINT('Ctrl Pts',(-1.05871835910697,-0.388086240756494,
-1.25722555095714));
#20235=CARTESIAN_POINT('Ctrl Pts',(-1.11153475808518,-0.407068917407805,
-1.2107812086231));
#20236=CARTESIAN_POINT('Ctrl Pts',(-1.13814686046673,-0.411552957311693,
-1.18575674747573));
#20237=CARTESIAN_POINT('Ctrl Pts',(-1.18575674747573,-0.411552957311693,
-1.13814686046673));
#20238=CARTESIAN_POINT('Ctrl Pts',(-1.2107812086231,-0.407068917407805,
-1.11153475808518));
#20239=CARTESIAN_POINT('Ctrl Pts',(-1.25722555095714,-0.388086240756494,
-1.05871835910697));
#20240=CARTESIAN_POINT('Ctrl Pts',(-1.27866649102984,-0.373586846396559,
-1.03253285680459));
#20241=CARTESIAN_POINT('Ctrl Pts',(-1.31521005565926,-0.33909093068465,
-0.985600426557816));
#20242=CARTESIAN_POINT('Ctrl Pts',(-1.33211611256184,-0.317195968905306,
-0.962485392528369));
#20243=CARTESIAN_POINT('Ctrl Pts',(-1.36127834356734,-0.266264900654909,
-0.920778333482565));
#20244=CARTESIAN_POINT('Ctrl Pts',(-1.3735491215176,-0.237231147975234,
-0.902193646979983));
#20245=CARTESIAN_POINT('Ctrl Pts',(-1.39550172959303,-0.166543350814306,
-0.867957148219442));
#20246=CARTESIAN_POINT('Ctrl Pts',(-1.40380622184538,-0.123401821157026,
-0.854205272175555));
#20247=CARTESIAN_POINT('Ctrl Pts',(-1.40825612658882,-0.07938,-0.846804978391753));
#20248=CARTESIAN_POINT('Origin',(-1.18440385848747,-0.07938,-1.18440385848747));
#20249=CARTESIAN_POINT('Origin',(0.,-0.07938,0.));
#20250=CARTESIAN_POINT('',(-0.397005914195118,-0.07938,-1.59456899932179));
#20251=CARTESIAN_POINT('Origin',(0.,-0.07938,0.));
#20252=CARTESIAN_POINT('Origin',(1.11022302462516E-16,-0.07938,-1.675));
#20253=CARTESIAN_POINT('Origin',(1.11022302462516E-16,0.,-1.675));
#20254=CARTESIAN_POINT('',(0.397005914195118,-0.07938,-1.59456899932179));
#20255=CARTESIAN_POINT('Ctrl Pts',(0.397005914195119,-0.0793800000000001,
-1.59456899932179));
#20256=CARTESIAN_POINT('Ctrl Pts',(0.388626558458099,-0.123401821157026,
-1.59665523941937));
#20257=CARTESIAN_POINT('Ctrl Pts',(0.373030350867485,-0.166543350814306,
-1.60050712143809));
#20258=CARTESIAN_POINT('Ctrl Pts',(0.333298652394954,-0.237231147975234,
-1.60919314384089));
#20259=CARTESIAN_POINT('Ctrl Pts',(0.311480544243686,-0.266264900654909,
-1.61365775139403));
#20260=CARTESIAN_POINT('Ctrl Pts',(0.261368388670537,-0.317195968905306,
-1.62252828437015));
#20261=CARTESIAN_POINT('Ctrl Pts',(0.233069203882014,-0.33909093068465,
-1.62691869420078));
#20262=CARTESIAN_POINT('Ctrl Pts',(0.174042761838763,-0.373586846396559,
-1.63426473152765));
#20263=CARTESIAN_POINT('Ctrl Pts',(0.140365781471549,-0.388086240756494,
-1.63761964365402));
#20264=CARTESIAN_POINT('Ctrl Pts',(0.0701778381840612,-0.407068917407805,
-1.64212536811722));
#20265=CARTESIAN_POINT('Ctrl Pts',(0.0336652739555916,-0.411552957311693,
-1.643248));
#20266=CARTESIAN_POINT('Ctrl Pts',(-0.0336652739555915,-0.411552957311693,
-1.643248));
#20267=CARTESIAN_POINT('Ctrl Pts',(-0.0701778381840612,-0.407068917407805,
-1.64212536811722));
#20268=CARTESIAN_POINT('Ctrl Pts',(-0.140365781471549,-0.388086240756494,
-1.63761964365402));
#20269=CARTESIAN_POINT('Ctrl Pts',(-0.174042761838764,-0.373586846396559,
-1.63426473152765));
#20270=CARTESIAN_POINT('Ctrl Pts',(-0.233069203882014,-0.33909093068465,
-1.62691869420078));
#20271=CARTESIAN_POINT('Ctrl Pts',(-0.261368388670536,-0.317195968905306,
-1.62252828437015));
#20272=CARTESIAN_POINT('Ctrl Pts',(-0.311480544243686,-0.266264900654908,
-1.61365775139403));
#20273=CARTESIAN_POINT('Ctrl Pts',(-0.333298652394954,-0.237231147975234,
-1.60919314384089));
#20274=CARTESIAN_POINT('Ctrl Pts',(-0.373030350867485,-0.166543350814306,
-1.60050712143809));
#20275=CARTESIAN_POINT('Ctrl Pts',(-0.388626558458099,-0.123401821157026,
-1.59665523941937));
#20276=CARTESIAN_POINT('Ctrl Pts',(-0.397005914195118,-0.07938,-1.59456899932179));
#20277=CARTESIAN_POINT('Origin',(1.11022302462516E-16,-0.07938,-1.675));
#20278=CARTESIAN_POINT('Origin',(0.,-0.07938,0.));
#20279=CARTESIAN_POINT('',(0.846804978391753,-0.07938,-1.40825612658882));
#20280=CARTESIAN_POINT('Origin',(0.,-0.07938,0.));
#20281=CARTESIAN_POINT('Origin',(1.18440385848747,-0.07938,-1.18440385848747));
#20282=CARTESIAN_POINT('Origin',(1.18440385848747,0.,-1.18440385848747));
#20283=CARTESIAN_POINT('',(1.40825612658882,-0.07938,-0.846804978391753));
#20284=CARTESIAN_POINT('Ctrl Pts',(1.40825612658882,-0.0793800000000001,
-0.846804978391753));
#20285=CARTESIAN_POINT('Ctrl Pts',(1.40380622184538,-0.123401821157026,
-0.854205272175555));
#20286=CARTESIAN_POINT('Ctrl Pts',(1.39550172959303,-0.166543350814306,
-0.867957148219442));
#20287=CARTESIAN_POINT('Ctrl Pts',(1.3735491215176,-0.237231147975234,-0.902193646979983));
#20288=CARTESIAN_POINT('Ctrl Pts',(1.36127834356734,-0.266264900654908,
-0.920778333482565));
#20289=CARTESIAN_POINT('Ctrl Pts',(1.33211611256184,-0.317195968905306,
-0.962485392528369));
#20290=CARTESIAN_POINT('Ctrl Pts',(1.31521005565926,-0.33909093068465,-0.985600426557816));
#20291=CARTESIAN_POINT('Ctrl Pts',(1.27866649102984,-0.373586846396559,
-1.03253285680459));
#20292=CARTESIAN_POINT('Ctrl Pts',(1.25722555095714,-0.388086240756494,
-1.05871835910697));
#20293=CARTESIAN_POINT('Ctrl Pts',(1.2107812086231,-0.407068917407805,-1.11153475808518));
#20294=CARTESIAN_POINT('Ctrl Pts',(1.18575674747573,-0.411552957311693,
-1.13814686046673));
#20295=CARTESIAN_POINT('Ctrl Pts',(1.13814686046673,-0.411552957311693,
-1.18575674747573));
#20296=CARTESIAN_POINT('Ctrl Pts',(1.11153475808518,-0.407068917407805,
-1.2107812086231));
#20297=CARTESIAN_POINT('Ctrl Pts',(1.05871835910697,-0.388086240756494,
-1.25722555095714));
#20298=CARTESIAN_POINT('Ctrl Pts',(1.03253285680459,-0.373586846396559,
-1.27866649102984));
#20299=CARTESIAN_POINT('Ctrl Pts',(0.985600426557816,-0.33909093068465,
-1.31521005565926));
#20300=CARTESIAN_POINT('Ctrl Pts',(0.962485392528369,-0.317195968905306,
-1.33211611256184));
#20301=CARTESIAN_POINT('Ctrl Pts',(0.920778333482565,-0.266264900654909,
-1.36127834356734));
#20302=CARTESIAN_POINT('Ctrl Pts',(0.902193646979983,-0.237231147975234,
-1.3735491215176));
#20303=CARTESIAN_POINT('Ctrl Pts',(0.867957148219442,-0.166543350814306,
-1.39550172959303));
#20304=CARTESIAN_POINT('Ctrl Pts',(0.854205272175555,-0.123401821157026,
-1.40380622184538));
#20305=CARTESIAN_POINT('Ctrl Pts',(0.846804978391753,-0.0793800000000001,
-1.40825612658882));
#20306=CARTESIAN_POINT('Origin',(1.18440385848747,-0.07938,-1.18440385848747));
#20307=CARTESIAN_POINT('Origin',(0.,-0.27783,0.));
#20308=CARTESIAN_POINT('',(-1.643248,-0.47628,2.01239840340529E-16));
#20309=CARTESIAN_POINT('Origin',(0.,-0.47628,0.));
#20310=CARTESIAN_POINT('',(-1.643248,-0.27783,2.01239840340529E-16));
#20311=CARTESIAN_POINT('',(1.59456899932179,-0.07938,0.397005914195118));
#20312=CARTESIAN_POINT('Origin',(0.,-0.07938,0.));
#20313=CARTESIAN_POINT('',(1.59456899932179,-0.07938,-0.397005914195118));
#20314=CARTESIAN_POINT('Ctrl Pts',(1.59456899932179,-0.0793800000000001,
0.397005914195118));
#20315=CARTESIAN_POINT('Ctrl Pts',(1.59665523941937,-0.123401821157026,
0.388626558458099));
#20316=CARTESIAN_POINT('Ctrl Pts',(1.60050712143809,-0.166543350814306,
0.373030350867485));
#20317=CARTESIAN_POINT('Ctrl Pts',(1.60919314384089,-0.237231147975234,
0.333298652394954));
#20318=CARTESIAN_POINT('Ctrl Pts',(1.61365775139403,-0.266264900654909,
0.311480544243686));
#20319=CARTESIAN_POINT('Ctrl Pts',(1.62252828437015,-0.317195968905306,
0.261368388670537));
#20320=CARTESIAN_POINT('Ctrl Pts',(1.62691869420078,-0.33909093068465,0.233069203882014));
#20321=CARTESIAN_POINT('Ctrl Pts',(1.63426473152765,-0.373586846396559,
0.174042761838764));
#20322=CARTESIAN_POINT('Ctrl Pts',(1.63761964365402,-0.388086240756494,
0.140365781471549));
#20323=CARTESIAN_POINT('Ctrl Pts',(1.64212536811722,-0.407068917407805,
0.0701778381840612));
#20324=CARTESIAN_POINT('Ctrl Pts',(1.643248,-0.411552957311693,0.0336652739555916));
#20325=CARTESIAN_POINT('Ctrl Pts',(1.643248,-0.411552957311693,-0.0336652739555916));
#20326=CARTESIAN_POINT('Ctrl Pts',(1.64212536811722,-0.407068917407805,
-0.0701778381840612));
#20327=CARTESIAN_POINT('Ctrl Pts',(1.63761964365402,-0.388086240756494,
-0.140365781471549));
#20328=CARTESIAN_POINT('Ctrl Pts',(1.63426473152765,-0.373586846396559,
-0.174042761838764));
#20329=CARTESIAN_POINT('Ctrl Pts',(1.62691869420078,-0.33909093068465,-0.233069203882014));
#20330=CARTESIAN_POINT('Ctrl Pts',(1.62252828437015,-0.317195968905306,
-0.261368388670537));
#20331=CARTESIAN_POINT('Ctrl Pts',(1.61365775139403,-0.266264900654909,
-0.311480544243686));
#20332=CARTESIAN_POINT('Ctrl Pts',(1.60919314384089,-0.237231147975234,
-0.333298652394954));
#20333=CARTESIAN_POINT('Ctrl Pts',(1.60050712143809,-0.166543350814306,
-0.373030350867485));
#20334=CARTESIAN_POINT('Ctrl Pts',(1.59665523941937,-0.123401821157026,
-0.388626558458099));
#20335=CARTESIAN_POINT('Ctrl Pts',(1.59456899932179,-0.07938,-0.397005914195118));
#20336=CARTESIAN_POINT('Origin',(0.,-0.07938,0.));
#20337=CARTESIAN_POINT('Origin',(0.,-0.07938,0.));
#20338=CARTESIAN_POINT('Origin',(1.675,-0.07938,0.));
#20339=CARTESIAN_POINT('Origin',(1.675,0.,0.));
#20340=CARTESIAN_POINT('Origin',(1.675,-0.07938,0.));
#20341=CARTESIAN_POINT('Origin',(0.,-0.47628,0.));
#20342=CARTESIAN_POINT('Origin',(0.,-0.07938,0.));
#33899=UNCERTAINTY_MEASURE_WITH_UNIT(LENGTH_MEASURE(0.001),#33982,
'DISTANCE_ACCURACY_VALUE',
'Maximum model space distance between geometric entities at asserted c
onnectivities');
#33929=UNCERTAINTY_MEASURE_WITH_UNIT(LENGTH_MEASURE(0.001),#33982,
'DISTANCE_ACCURACY_VALUE',
'Maximum model space distance between geometric entities at asserted c
onnectivities');
#33951=(
GEOMETRIC_REPRESENTATION_CONTEXT(3)
GLOBAL_UNCERTAINTY_ASSIGNED_CONTEXT((#33899))
GLOBAL_UNIT_ASSIGNED_CONTEXT((#33982,#33984,#33985))
REPRESENTATION_CONTEXT('','3D')
);
#33981=(
GEOMETRIC_REPRESENTATION_CONTEXT(3)
GLOBAL_UNCERTAINTY_ASSIGNED_CONTEXT((#33929))
GLOBAL_UNIT_ASSIGNED_CONTEXT((#33982,#33984,#33985))
REPRESENTATION_CONTEXT('','3D')
);
#33982=(
LENGTH_UNIT()
NAMED_UNIT(*)
SI_UNIT(.CENTI.,.METRE.)
);
#33984=(
NAMED_UNIT(*)
PLANE_ANGLE_UNIT()
SI_UNIT($,.RADIAN.)
);
#33985=(
NAMED_UNIT(*)
SI_UNIT($,.STERADIAN.)
SOLID_ANGLE_UNIT()
);
#34007=SHAPE_DEFINITION_REPRESENTATION(#34063,#34203);
#34063=PRODUCT_DEFINITION_SHAPE('',$,#34255);
#34203=SHAPE_REPRESENTATION('',(#14057),#33951);
#34233=PRODUCT_DEFINITION_CONTEXT('part definition',#34388,'design');
#34255=PRODUCT_DEFINITION('Cage (1)','Cage (1)',#34306,#34233);
#34306=PRODUCT_DEFINITION_FORMATION('',$,#34411);
#34388=APPLICATION_CONTEXT(
'Core Data for Automotive Mechanical Design Process');
#34389=PRODUCT_CONTEXT('part definition',#34388,'mechanical');
#34411=PRODUCT('Cage (1)','Cage (1)','Cage (1)',(#34389));
#34511=COLOUR_RGB('Grey',0.48,0.52,0.57);
#34512=FILL_AREA_STYLE_COLOUR('',#34511);
#34513=FILL_AREA_STYLE('',(#34512));
#34514=SURFACE_STYLE_FILL_AREA(#34513);
#34515=SURFACE_SIDE_STYLE('',(#34514));
#34516=SURFACE_STYLE_USAGE(.BOTH.,#34515);
#34517=PRESENTATION_STYLE_ASSIGNMENT((#34516));
ENDSEC;
END-ISO-10303-21;
